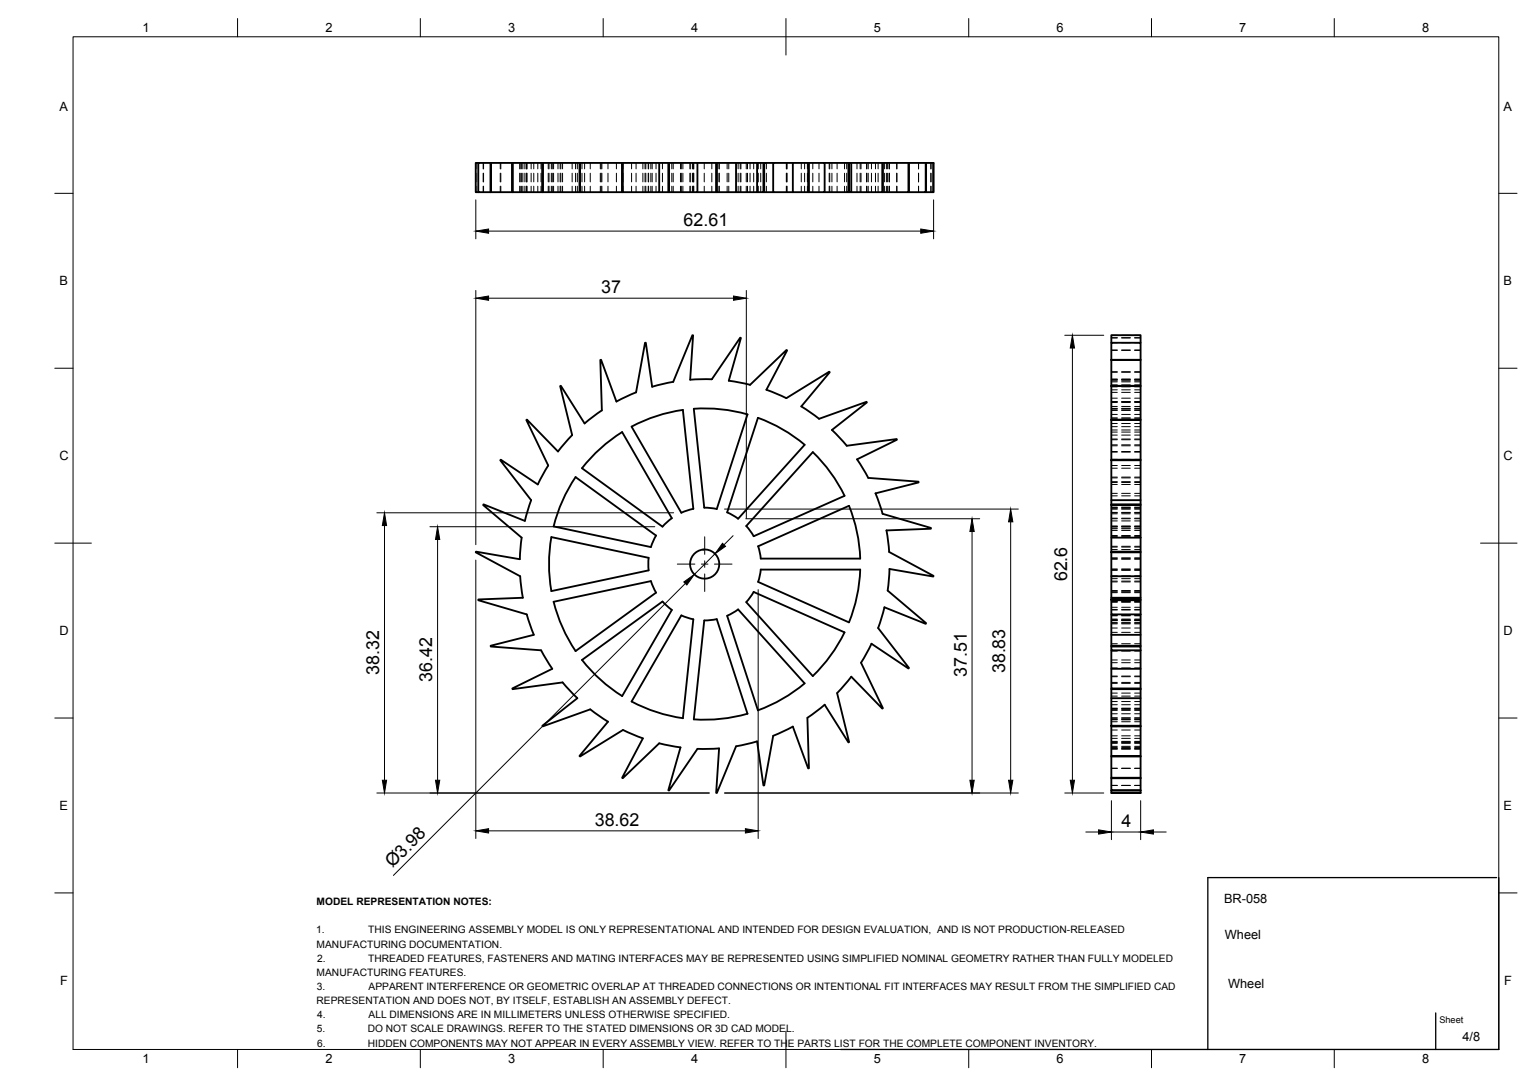
ISO-10303-21;
HEADER;
/* Generated by software containing ST-Developer
 * from STEP Tools, Inc. (www.steptools.com) 
 */

FILE_DESCRIPTION(
/* description */ (''),
/* implementation_level */ '2;1');

FILE_NAME(
/* name */ 'Wheel.step',
/* time_stamp */ '2026-10-12T16:07:47-07:00',
/* author */ (''),
/* organization */ (''),
/* preprocessor_version */ 'ST-DEVELOPER v20.2',
/* originating_system */ 'Autodesk Translation Framework v15.15.0.0',
/* authorisation */ '');

FILE_SCHEMA (('AUTOMOTIVE_DESIGN { 1 0 10303 214 3 1 1 }'));
ENDSEC;

DATA;
#10=MECHANICAL_DESIGN_GEOMETRIC_PRESENTATION_REPRESENTATION('',(#94),#8779);
#80=SHAPE_REPRESENTATION_RELATIONSHIP('SRR','None',#8809,#87);
#87=ADVANCED_BREP_SHAPE_REPRESENTATION('',(#104),#8772);
#94=STYLED_ITEM('',(#8853),#104);
#104=MANIFOLD_SOLID_BREP('Body1',#5114);
#114=FACE_BOUND('',#934,.T.);
#115=FACE_BOUND('',#935,.T.);
#116=FACE_BOUND('',#936,.T.);
#117=FACE_BOUND('',#937,.T.);
#118=FACE_BOUND('',#938,.T.);
#119=FACE_BOUND('',#939,.T.);
#120=FACE_BOUND('',#940,.T.);
#121=FACE_BOUND('',#941,.T.);
#122=FACE_BOUND('',#942,.T.);
#123=FACE_BOUND('',#943,.T.);
#124=FACE_BOUND('',#944,.T.);
#125=FACE_BOUND('',#945,.T.);
#126=FACE_BOUND('',#946,.T.);
#127=FACE_BOUND('',#947,.T.);
#128=FACE_BOUND('',#948,.T.);
#129=FACE_BOUND('',#949,.T.);
#130=FACE_BOUND('',#951,.T.);
#131=FACE_BOUND('',#952,.T.);
#132=FACE_BOUND('',#953,.T.);
#133=FACE_BOUND('',#954,.T.);
#134=FACE_BOUND('',#955,.T.);
#135=FACE_BOUND('',#956,.T.);
#136=FACE_BOUND('',#957,.T.);
#137=FACE_BOUND('',#958,.T.);
#138=FACE_BOUND('',#959,.T.);
#139=FACE_BOUND('',#960,.T.);
#140=FACE_BOUND('',#961,.T.);
#141=FACE_BOUND('',#962,.T.);
#142=FACE_BOUND('',#963,.T.);
#143=FACE_BOUND('',#964,.T.);
#144=FACE_BOUND('',#965,.T.);
#145=FACE_BOUND('',#966,.T.);
#169=CIRCLE('',#5208,25.2882678496568);
#170=CIRCLE('',#5209,25.2882678496568);
#171=CIRCLE('',#5211,25.2882678496568);
#172=CIRCLE('',#5212,25.2882678496568);
#173=CIRCLE('',#5217,25.2882678496568);
#174=CIRCLE('',#5218,25.2882678496568);
#175=CIRCLE('',#5220,25.2882678496568);
#176=CIRCLE('',#5221,25.2882678496568);
#177=CIRCLE('',#5226,25.2882678496568);
#178=CIRCLE('',#5227,25.2882678496568);
#179=CIRCLE('',#5232,25.2882678496568);
#180=CIRCLE('',#5233,25.2882678496568);
#181=CIRCLE('',#5235,25.2882678496568);
#182=CIRCLE('',#5236,25.2882678496568);
#183=CIRCLE('',#5244,25.2882678496568);
#184=CIRCLE('',#5245,25.2882678496568);
#185=CIRCLE('',#5250,25.2882678496568);
#186=CIRCLE('',#5251,25.2882678496568);
#187=CIRCLE('',#5258,21.2882678496568);
#188=CIRCLE('',#5259,21.2882678496568);
#189=CIRCLE('',#5261,21.2882678496568);
#190=CIRCLE('',#5262,21.2882678496568);
#191=CIRCLE('',#5264,7.71108476483471);
#192=CIRCLE('',#5265,7.71108476483471);
#193=CIRCLE('',#5267,7.71108476483471);
#194=CIRCLE('',#5268,7.71108476483471);
#195=CIRCLE('',#5272,21.2882678496568);
#196=CIRCLE('',#5273,21.2882678496568);
#197=CIRCLE('',#5275,7.71108476483471);
#198=CIRCLE('',#5276,7.71108476483471);
#199=CIRCLE('',#5280,21.2882678496568);
#200=CIRCLE('',#5281,21.2882678496568);
#201=CIRCLE('',#5283,7.71108476483471);
#202=CIRCLE('',#5284,7.71108476483471);
#203=CIRCLE('',#5289,25.2882678496568);
#204=CIRCLE('',#5290,25.2882678496568);
#205=CIRCLE('',#5292,25.2882678496568);
#206=CIRCLE('',#5293,25.2882678496568);
#207=CIRCLE('',#5298,25.2882678496568);
#208=CIRCLE('',#5299,25.2882678496568);
#209=CIRCLE('',#5301,25.2882678496568);
#210=CIRCLE('',#5302,25.2882678496568);
#211=CIRCLE('',#5307,25.2882678496568);
#212=CIRCLE('',#5308,25.2882678496568);
#213=CIRCLE('',#5316,25.2882678496568);
#214=CIRCLE('',#5317,25.2882678496568);
#215=CIRCLE('',#5324,21.2882678496568);
#216=CIRCLE('',#5325,21.2882678496568);
#217=CIRCLE('',#5327,21.2882678496568);
#218=CIRCLE('',#5328,21.2882678496568);
#219=CIRCLE('',#5330,7.71108476483471);
#220=CIRCLE('',#5331,7.71108476483471);
#221=CIRCLE('',#5333,7.71108476483471);
#222=CIRCLE('',#5334,7.71108476483471);
#223=CIRCLE('',#5338,21.2882678496568);
#224=CIRCLE('',#5339,21.2882678496568);
#225=CIRCLE('',#5341,7.71108476483471);
#226=CIRCLE('',#5342,7.71108476483471);
#227=CIRCLE('',#5346,21.2882678496568);
#228=CIRCLE('',#5347,21.2882678496568);
#229=CIRCLE('',#5349,21.2882678496568);
#230=CIRCLE('',#5350,21.2882678496568);
#231=CIRCLE('',#5352,7.71108476483471);
#232=CIRCLE('',#5353,7.71108476483471);
#233=CIRCLE('',#5355,7.71108476483471);
#234=CIRCLE('',#5356,7.71108476483471);
#235=CIRCLE('',#5360,21.2882678496568);
#236=CIRCLE('',#5361,21.2882678496568);
#237=CIRCLE('',#5363,21.2882678496568);
#238=CIRCLE('',#5364,21.2882678496568);
#239=CIRCLE('',#5366,7.71108476483471);
#240=CIRCLE('',#5367,7.71108476483471);
#241=CIRCLE('',#5369,7.71108476483471);
#242=CIRCLE('',#5370,7.71108476483471);
#243=CIRCLE('',#5374,21.2882678496568);
#244=CIRCLE('',#5375,21.2882678496568);
#245=CIRCLE('',#5377,7.71108476483471);
#246=CIRCLE('',#5378,7.71108476483471);
#247=CIRCLE('',#5384,21.2882678496568);
#248=CIRCLE('',#5385,21.2882678496568);
#249=CIRCLE('',#5387,7.71108476483471);
#250=CIRCLE('',#5388,7.71108476483471);
#251=CIRCLE('',#5395,25.2882678496568);
#252=CIRCLE('',#5396,25.2882678496568);
#253=CIRCLE('',#5398,25.2882678496568);
#254=CIRCLE('',#5399,25.2882678496568);
#255=CIRCLE('',#5404,25.2882678496568);
#256=CIRCLE('',#5405,25.2882678496568);
#257=CIRCLE('',#5410,25.2882678496568);
#258=CIRCLE('',#5411,25.2882678496568);
#259=CIRCLE('',#5413,25.2882678496568);
#260=CIRCLE('',#5414,25.2882678496568);
#261=CIRCLE('',#5419,25.2882678496568);
#262=CIRCLE('',#5420,25.2882678496568);
#263=CIRCLE('',#5422,25.2882678496568);
#264=CIRCLE('',#5423,25.2882678496568);
#265=CIRCLE('',#5437,25.2882678496568);
#266=CIRCLE('',#5438,25.2882678496568);
#267=CIRCLE('',#5442,21.2882678496568);
#268=CIRCLE('',#5443,21.2882678496568);
#269=CIRCLE('',#5445,7.71108476483471);
#270=CIRCLE('',#5446,7.71108476483471);
#271=CIRCLE('',#5450,21.2882678496568);
#272=CIRCLE('',#5451,21.2882678496568);
#273=CIRCLE('',#5453,7.71108476483471);
#274=CIRCLE('',#5454,7.71108476483471);
#275=CIRCLE('',#5461,25.2882678496568);
#276=CIRCLE('',#5462,25.2882678496568);
#277=CIRCLE('',#5464,25.2882678496568);
#278=CIRCLE('',#5465,25.2882678496568);
#279=CIRCLE('',#5470,25.2882678496568);
#280=CIRCLE('',#5471,25.2882678496568);
#281=CIRCLE('',#5476,25.2882678496568);
#282=CIRCLE('',#5477,25.2882678496568);
#283=CIRCLE('',#5479,25.2882678496568);
#284=CIRCLE('',#5480,25.2882678496568);
#285=CIRCLE('',#5485,25.2882678496568);
#286=CIRCLE('',#5486,25.2882678496568);
#287=CIRCLE('',#5491,25.2882678496568);
#288=CIRCLE('',#5492,25.2882678496568);
#289=CIRCLE('',#5505,1.99137169252308);
#290=CIRCLE('',#5506,1.99137169252308);
#396=CYLINDRICAL_SURFACE('',#5207,25.2882678496568);
#397=CYLINDRICAL_SURFACE('',#5210,25.2882678496568);
#398=CYLINDRICAL_SURFACE('',#5216,25.2882678496568);
#399=CYLINDRICAL_SURFACE('',#5219,25.2882678496568);
#400=CYLINDRICAL_SURFACE('',#5225,25.2882678496568);
#401=CYLINDRICAL_SURFACE('',#5231,25.2882678496568);
#402=CYLINDRICAL_SURFACE('',#5234,25.2882678496568);
#403=CYLINDRICAL_SURFACE('',#5243,25.2882678496568);
#404=CYLINDRICAL_SURFACE('',#5249,25.2882678496568);
#405=CYLINDRICAL_SURFACE('',#5257,21.2882678496568);
#406=CYLINDRICAL_SURFACE('',#5260,21.2882678496568);
#407=CYLINDRICAL_SURFACE('',#5263,7.71108476483471);
#408=CYLINDRICAL_SURFACE('',#5266,7.71108476483471);
#409=CYLINDRICAL_SURFACE('',#5271,21.2882678496568);
#410=CYLINDRICAL_SURFACE('',#5274,7.71108476483471);
#411=CYLINDRICAL_SURFACE('',#5279,21.2882678496568);
#412=CYLINDRICAL_SURFACE('',#5282,7.71108476483471);
#413=CYLINDRICAL_SURFACE('',#5288,25.2882678496568);
#414=CYLINDRICAL_SURFACE('',#5291,25.2882678496568);
#415=CYLINDRICAL_SURFACE('',#5297,25.2882678496568);
#416=CYLINDRICAL_SURFACE('',#5300,25.2882678496568);
#417=CYLINDRICAL_SURFACE('',#5306,25.2882678496568);
#418=CYLINDRICAL_SURFACE('',#5315,25.2882678496568);
#419=CYLINDRICAL_SURFACE('',#5323,21.2882678496568);
#420=CYLINDRICAL_SURFACE('',#5326,21.2882678496568);
#421=CYLINDRICAL_SURFACE('',#5329,7.71108476483471);
#422=CYLINDRICAL_SURFACE('',#5332,7.71108476483471);
#423=CYLINDRICAL_SURFACE('',#5337,21.2882678496568);
#424=CYLINDRICAL_SURFACE('',#5340,7.71108476483471);
#425=CYLINDRICAL_SURFACE('',#5345,21.2882678496568);
#426=CYLINDRICAL_SURFACE('',#5348,21.2882678496568);
#427=CYLINDRICAL_SURFACE('',#5351,7.71108476483471);
#428=CYLINDRICAL_SURFACE('',#5354,7.71108476483471);
#429=CYLINDRICAL_SURFACE('',#5359,21.2882678496568);
#430=CYLINDRICAL_SURFACE('',#5362,21.2882678496568);
#431=CYLINDRICAL_SURFACE('',#5365,7.71108476483471);
#432=CYLINDRICAL_SURFACE('',#5368,7.71108476483471);
#433=CYLINDRICAL_SURFACE('',#5373,21.2882678496568);
#434=CYLINDRICAL_SURFACE('',#5376,7.71108476483471);
#435=CYLINDRICAL_SURFACE('',#5383,21.2882678496568);
#436=CYLINDRICAL_SURFACE('',#5386,7.71108476483471);
#437=CYLINDRICAL_SURFACE('',#5394,25.2882678496568);
#438=CYLINDRICAL_SURFACE('',#5397,25.2882678496568);
#439=CYLINDRICAL_SURFACE('',#5403,25.2882678496568);
#440=CYLINDRICAL_SURFACE('',#5409,25.2882678496568);
#441=CYLINDRICAL_SURFACE('',#5412,25.2882678496568);
#442=CYLINDRICAL_SURFACE('',#5418,25.2882678496568);
#443=CYLINDRICAL_SURFACE('',#5421,25.2882678496568);
#444=CYLINDRICAL_SURFACE('',#5436,25.2882678496568);
#445=CYLINDRICAL_SURFACE('',#5441,21.2882678496568);
#446=CYLINDRICAL_SURFACE('',#5444,7.71108476483471);
#447=CYLINDRICAL_SURFACE('',#5449,21.2882678496568);
#448=CYLINDRICAL_SURFACE('',#5452,7.71108476483471);
#449=CYLINDRICAL_SURFACE('',#5460,25.2882678496568);
#450=CYLINDRICAL_SURFACE('',#5463,25.2882678496568);
#451=CYLINDRICAL_SURFACE('',#5469,25.2882678496568);
#452=CYLINDRICAL_SURFACE('',#5475,25.2882678496568);
#453=CYLINDRICAL_SURFACE('',#5478,25.2882678496568);
#454=CYLINDRICAL_SURFACE('',#5484,25.2882678496568);
#455=CYLINDRICAL_SURFACE('',#5490,25.2882678496568);
#456=CYLINDRICAL_SURFACE('',#5504,1.99137169252308);
#475=FACE_OUTER_BOUND('',#752,.T.);
#476=FACE_OUTER_BOUND('',#753,.T.);
#477=FACE_OUTER_BOUND('',#754,.T.);
#478=FACE_OUTER_BOUND('',#755,.T.);
#479=FACE_OUTER_BOUND('',#756,.T.);
#480=FACE_OUTER_BOUND('',#757,.T.);
#481=FACE_OUTER_BOUND('',#758,.T.);
#482=FACE_OUTER_BOUND('',#759,.T.);
#483=FACE_OUTER_BOUND('',#760,.T.);
#484=FACE_OUTER_BOUND('',#761,.T.);
#485=FACE_OUTER_BOUND('',#762,.T.);
#486=FACE_OUTER_BOUND('',#763,.T.);
#487=FACE_OUTER_BOUND('',#764,.T.);
#488=FACE_OUTER_BOUND('',#765,.T.);
#489=FACE_OUTER_BOUND('',#766,.T.);
#490=FACE_OUTER_BOUND('',#767,.T.);
#491=FACE_OUTER_BOUND('',#768,.T.);
#492=FACE_OUTER_BOUND('',#769,.T.);
#493=FACE_OUTER_BOUND('',#770,.T.);
#494=FACE_OUTER_BOUND('',#771,.T.);
#495=FACE_OUTER_BOUND('',#772,.T.);
#496=FACE_OUTER_BOUND('',#773,.T.);
#497=FACE_OUTER_BOUND('',#774,.T.);
#498=FACE_OUTER_BOUND('',#775,.T.);
#499=FACE_OUTER_BOUND('',#776,.T.);
#500=FACE_OUTER_BOUND('',#777,.T.);
#501=FACE_OUTER_BOUND('',#778,.T.);
#502=FACE_OUTER_BOUND('',#779,.T.);
#503=FACE_OUTER_BOUND('',#780,.T.);
#504=FACE_OUTER_BOUND('',#781,.T.);
#505=FACE_OUTER_BOUND('',#782,.T.);
#506=FACE_OUTER_BOUND('',#783,.T.);
#507=FACE_OUTER_BOUND('',#784,.T.);
#508=FACE_OUTER_BOUND('',#785,.T.);
#509=FACE_OUTER_BOUND('',#786,.T.);
#510=FACE_OUTER_BOUND('',#787,.T.);
#511=FACE_OUTER_BOUND('',#788,.T.);
#512=FACE_OUTER_BOUND('',#789,.T.);
#513=FACE_OUTER_BOUND('',#790,.T.);
#514=FACE_OUTER_BOUND('',#791,.T.);
#515=FACE_OUTER_BOUND('',#792,.T.);
#516=FACE_OUTER_BOUND('',#793,.T.);
#517=FACE_OUTER_BOUND('',#794,.T.);
#518=FACE_OUTER_BOUND('',#795,.T.);
#519=FACE_OUTER_BOUND('',#796,.T.);
#520=FACE_OUTER_BOUND('',#797,.T.);
#521=FACE_OUTER_BOUND('',#798,.T.);
#522=FACE_OUTER_BOUND('',#799,.T.);
#523=FACE_OUTER_BOUND('',#800,.T.);
#524=FACE_OUTER_BOUND('',#801,.T.);
#525=FACE_OUTER_BOUND('',#802,.T.);
#526=FACE_OUTER_BOUND('',#803,.T.);
#527=FACE_OUTER_BOUND('',#804,.T.);
#528=FACE_OUTER_BOUND('',#805,.T.);
#529=FACE_OUTER_BOUND('',#806,.T.);
#530=FACE_OUTER_BOUND('',#807,.T.);
#531=FACE_OUTER_BOUND('',#808,.T.);
#532=FACE_OUTER_BOUND('',#809,.T.);
#533=FACE_OUTER_BOUND('',#810,.T.);
#534=FACE_OUTER_BOUND('',#811,.T.);
#535=FACE_OUTER_BOUND('',#812,.T.);
#536=FACE_OUTER_BOUND('',#813,.T.);
#537=FACE_OUTER_BOUND('',#814,.T.);
#538=FACE_OUTER_BOUND('',#815,.T.);
#539=FACE_OUTER_BOUND('',#816,.T.);
#540=FACE_OUTER_BOUND('',#817,.T.);
#541=FACE_OUTER_BOUND('',#818,.T.);
#542=FACE_OUTER_BOUND('',#819,.T.);
#543=FACE_OUTER_BOUND('',#820,.T.);
#544=FACE_OUTER_BOUND('',#821,.T.);
#545=FACE_OUTER_BOUND('',#822,.T.);
#546=FACE_OUTER_BOUND('',#823,.T.);
#547=FACE_OUTER_BOUND('',#824,.T.);
#548=FACE_OUTER_BOUND('',#825,.T.);
#549=FACE_OUTER_BOUND('',#826,.T.);
#550=FACE_OUTER_BOUND('',#827,.T.);
#551=FACE_OUTER_BOUND('',#828,.T.);
#552=FACE_OUTER_BOUND('',#829,.T.);
#553=FACE_OUTER_BOUND('',#830,.T.);
#554=FACE_OUTER_BOUND('',#831,.T.);
#555=FACE_OUTER_BOUND('',#832,.T.);
#556=FACE_OUTER_BOUND('',#833,.T.);
#557=FACE_OUTER_BOUND('',#834,.T.);
#558=FACE_OUTER_BOUND('',#835,.T.);
#559=FACE_OUTER_BOUND('',#836,.T.);
#560=FACE_OUTER_BOUND('',#837,.T.);
#561=FACE_OUTER_BOUND('',#838,.T.);
#562=FACE_OUTER_BOUND('',#839,.T.);
#563=FACE_OUTER_BOUND('',#840,.T.);
#564=FACE_OUTER_BOUND('',#841,.T.);
#565=FACE_OUTER_BOUND('',#842,.T.);
#566=FACE_OUTER_BOUND('',#843,.T.);
#567=FACE_OUTER_BOUND('',#844,.T.);
#568=FACE_OUTER_BOUND('',#845,.T.);
#569=FACE_OUTER_BOUND('',#846,.T.);
#570=FACE_OUTER_BOUND('',#847,.T.);
#571=FACE_OUTER_BOUND('',#848,.T.);
#572=FACE_OUTER_BOUND('',#849,.T.);
#573=FACE_OUTER_BOUND('',#850,.T.);
#574=FACE_OUTER_BOUND('',#851,.T.);
#575=FACE_OUTER_BOUND('',#852,.T.);
#576=FACE_OUTER_BOUND('',#853,.T.);
#577=FACE_OUTER_BOUND('',#854,.T.);
#578=FACE_OUTER_BOUND('',#855,.T.);
#579=FACE_OUTER_BOUND('',#856,.T.);
#580=FACE_OUTER_BOUND('',#857,.T.);
#581=FACE_OUTER_BOUND('',#858,.T.);
#582=FACE_OUTER_BOUND('',#859,.T.);
#583=FACE_OUTER_BOUND('',#860,.T.);
#584=FACE_OUTER_BOUND('',#861,.T.);
#585=FACE_OUTER_BOUND('',#862,.T.);
#586=FACE_OUTER_BOUND('',#863,.T.);
#587=FACE_OUTER_BOUND('',#864,.T.);
#588=FACE_OUTER_BOUND('',#865,.T.);
#589=FACE_OUTER_BOUND('',#866,.T.);
#590=FACE_OUTER_BOUND('',#867,.T.);
#591=FACE_OUTER_BOUND('',#868,.T.);
#592=FACE_OUTER_BOUND('',#869,.T.);
#593=FACE_OUTER_BOUND('',#870,.T.);
#594=FACE_OUTER_BOUND('',#871,.T.);
#595=FACE_OUTER_BOUND('',#872,.T.);
#596=FACE_OUTER_BOUND('',#873,.T.);
#597=FACE_OUTER_BOUND('',#874,.T.);
#598=FACE_OUTER_BOUND('',#875,.T.);
#599=FACE_OUTER_BOUND('',#876,.T.);
#600=FACE_OUTER_BOUND('',#877,.T.);
#601=FACE_OUTER_BOUND('',#878,.T.);
#602=FACE_OUTER_BOUND('',#879,.T.);
#603=FACE_OUTER_BOUND('',#880,.T.);
#604=FACE_OUTER_BOUND('',#881,.T.);
#605=FACE_OUTER_BOUND('',#882,.T.);
#606=FACE_OUTER_BOUND('',#883,.T.);
#607=FACE_OUTER_BOUND('',#884,.T.);
#608=FACE_OUTER_BOUND('',#885,.T.);
#609=FACE_OUTER_BOUND('',#886,.T.);
#610=FACE_OUTER_BOUND('',#887,.T.);
#611=FACE_OUTER_BOUND('',#888,.T.);
#612=FACE_OUTER_BOUND('',#889,.T.);
#613=FACE_OUTER_BOUND('',#890,.T.);
#614=FACE_OUTER_BOUND('',#891,.T.);
#615=FACE_OUTER_BOUND('',#892,.T.);
#616=FACE_OUTER_BOUND('',#893,.T.);
#617=FACE_OUTER_BOUND('',#894,.T.);
#618=FACE_OUTER_BOUND('',#895,.T.);
#619=FACE_OUTER_BOUND('',#896,.T.);
#620=FACE_OUTER_BOUND('',#897,.T.);
#621=FACE_OUTER_BOUND('',#898,.T.);
#622=FACE_OUTER_BOUND('',#899,.T.);
#623=FACE_OUTER_BOUND('',#900,.T.);
#624=FACE_OUTER_BOUND('',#901,.T.);
#625=FACE_OUTER_BOUND('',#902,.T.);
#626=FACE_OUTER_BOUND('',#903,.T.);
#627=FACE_OUTER_BOUND('',#904,.T.);
#628=FACE_OUTER_BOUND('',#905,.T.);
#629=FACE_OUTER_BOUND('',#906,.T.);
#630=FACE_OUTER_BOUND('',#907,.T.);
#631=FACE_OUTER_BOUND('',#908,.T.);
#632=FACE_OUTER_BOUND('',#909,.T.);
#633=FACE_OUTER_BOUND('',#910,.T.);
#634=FACE_OUTER_BOUND('',#911,.T.);
#635=FACE_OUTER_BOUND('',#912,.T.);
#636=FACE_OUTER_BOUND('',#913,.T.);
#637=FACE_OUTER_BOUND('',#914,.T.);
#638=FACE_OUTER_BOUND('',#915,.T.);
#639=FACE_OUTER_BOUND('',#916,.T.);
#640=FACE_OUTER_BOUND('',#917,.T.);
#641=FACE_OUTER_BOUND('',#918,.T.);
#642=FACE_OUTER_BOUND('',#919,.T.);
#643=FACE_OUTER_BOUND('',#920,.T.);
#644=FACE_OUTER_BOUND('',#921,.T.);
#645=FACE_OUTER_BOUND('',#922,.T.);
#646=FACE_OUTER_BOUND('',#923,.T.);
#647=FACE_OUTER_BOUND('',#924,.T.);
#648=FACE_OUTER_BOUND('',#925,.T.);
#649=FACE_OUTER_BOUND('',#926,.T.);
#650=FACE_OUTER_BOUND('',#927,.T.);
#651=FACE_OUTER_BOUND('',#928,.T.);
#652=FACE_OUTER_BOUND('',#929,.T.);
#653=FACE_OUTER_BOUND('',#930,.T.);
#654=FACE_OUTER_BOUND('',#931,.T.);
#655=FACE_OUTER_BOUND('',#932,.T.);
#656=FACE_OUTER_BOUND('',#933,.T.);
#657=FACE_OUTER_BOUND('',#950,.T.);
#752=EDGE_LOOP('',(#3240,#3241,#3242,#3243));
#753=EDGE_LOOP('',(#3244,#3245,#3246,#3247));
#754=EDGE_LOOP('',(#3248,#3249,#3250,#3251));
#755=EDGE_LOOP('',(#3252,#3253,#3254,#3255));
#756=EDGE_LOOP('',(#3256,#3257,#3258,#3259));
#757=EDGE_LOOP('',(#3260,#3261,#3262,#3263));
#758=EDGE_LOOP('',(#3264,#3265,#3266,#3267));
#759=EDGE_LOOP('',(#3268,#3269,#3270,#3271));
#760=EDGE_LOOP('',(#3272,#3273,#3274,#3275));
#761=EDGE_LOOP('',(#3276,#3277,#3278,#3279));
#762=EDGE_LOOP('',(#3280,#3281,#3282,#3283));
#763=EDGE_LOOP('',(#3284,#3285,#3286,#3287));
#764=EDGE_LOOP('',(#3288,#3289,#3290,#3291));
#765=EDGE_LOOP('',(#3292,#3293,#3294,#3295));
#766=EDGE_LOOP('',(#3296,#3297,#3298,#3299));
#767=EDGE_LOOP('',(#3300,#3301,#3302,#3303));
#768=EDGE_LOOP('',(#3304,#3305,#3306,#3307));
#769=EDGE_LOOP('',(#3308,#3309,#3310,#3311));
#770=EDGE_LOOP('',(#3312,#3313,#3314,#3315));
#771=EDGE_LOOP('',(#3316,#3317,#3318,#3319));
#772=EDGE_LOOP('',(#3320,#3321,#3322,#3323));
#773=EDGE_LOOP('',(#3324,#3325,#3326,#3327));
#774=EDGE_LOOP('',(#3328,#3329,#3330,#3331));
#775=EDGE_LOOP('',(#3332,#3333,#3334,#3335));
#776=EDGE_LOOP('',(#3336,#3337,#3338,#3339));
#777=EDGE_LOOP('',(#3340,#3341,#3342,#3343));
#778=EDGE_LOOP('',(#3344,#3345,#3346,#3347));
#779=EDGE_LOOP('',(#3348,#3349,#3350,#3351));
#780=EDGE_LOOP('',(#3352,#3353,#3354,#3355));
#781=EDGE_LOOP('',(#3356,#3357,#3358,#3359));
#782=EDGE_LOOP('',(#3360,#3361,#3362,#3363));
#783=EDGE_LOOP('',(#3364,#3365,#3366,#3367));
#784=EDGE_LOOP('',(#3368,#3369,#3370,#3371));
#785=EDGE_LOOP('',(#3372,#3373,#3374,#3375));
#786=EDGE_LOOP('',(#3376,#3377,#3378,#3379));
#787=EDGE_LOOP('',(#3380,#3381,#3382,#3383));
#788=EDGE_LOOP('',(#3384,#3385,#3386,#3387));
#789=EDGE_LOOP('',(#3388,#3389,#3390,#3391));
#790=EDGE_LOOP('',(#3392,#3393,#3394,#3395));
#791=EDGE_LOOP('',(#3396,#3397,#3398,#3399));
#792=EDGE_LOOP('',(#3400,#3401,#3402,#3403));
#793=EDGE_LOOP('',(#3404,#3405,#3406,#3407));
#794=EDGE_LOOP('',(#3408,#3409,#3410,#3411));
#795=EDGE_LOOP('',(#3412,#3413,#3414,#3415));
#796=EDGE_LOOP('',(#3416,#3417,#3418,#3419));
#797=EDGE_LOOP('',(#3420,#3421,#3422,#3423));
#798=EDGE_LOOP('',(#3424,#3425,#3426,#3427));
#799=EDGE_LOOP('',(#3428,#3429,#3430,#3431));
#800=EDGE_LOOP('',(#3432,#3433,#3434,#3435));
#801=EDGE_LOOP('',(#3436,#3437,#3438,#3439));
#802=EDGE_LOOP('',(#3440,#3441,#3442,#3443));
#803=EDGE_LOOP('',(#3444,#3445,#3446,#3447));
#804=EDGE_LOOP('',(#3448,#3449,#3450,#3451));
#805=EDGE_LOOP('',(#3452,#3453,#3454,#3455));
#806=EDGE_LOOP('',(#3456,#3457,#3458,#3459));
#807=EDGE_LOOP('',(#3460,#3461,#3462,#3463));
#808=EDGE_LOOP('',(#3464,#3465,#3466,#3467));
#809=EDGE_LOOP('',(#3468,#3469,#3470,#3471));
#810=EDGE_LOOP('',(#3472,#3473,#3474,#3475));
#811=EDGE_LOOP('',(#3476,#3477,#3478,#3479));
#812=EDGE_LOOP('',(#3480,#3481,#3482,#3483));
#813=EDGE_LOOP('',(#3484,#3485,#3486,#3487));
#814=EDGE_LOOP('',(#3488,#3489,#3490,#3491));
#815=EDGE_LOOP('',(#3492,#3493,#3494,#3495));
#816=EDGE_LOOP('',(#3496,#3497,#3498,#3499));
#817=EDGE_LOOP('',(#3500,#3501,#3502,#3503));
#818=EDGE_LOOP('',(#3504,#3505,#3506,#3507));
#819=EDGE_LOOP('',(#3508,#3509,#3510,#3511));
#820=EDGE_LOOP('',(#3512,#3513,#3514,#3515));
#821=EDGE_LOOP('',(#3516,#3517,#3518,#3519));
#822=EDGE_LOOP('',(#3520,#3521,#3522,#3523));
#823=EDGE_LOOP('',(#3524,#3525,#3526,#3527));
#824=EDGE_LOOP('',(#3528,#3529,#3530,#3531));
#825=EDGE_LOOP('',(#3532,#3533,#3534,#3535));
#826=EDGE_LOOP('',(#3536,#3537,#3538,#3539));
#827=EDGE_LOOP('',(#3540,#3541,#3542,#3543));
#828=EDGE_LOOP('',(#3544,#3545,#3546,#3547));
#829=EDGE_LOOP('',(#3548,#3549,#3550,#3551));
#830=EDGE_LOOP('',(#3552,#3553,#3554,#3555));
#831=EDGE_LOOP('',(#3556,#3557,#3558,#3559));
#832=EDGE_LOOP('',(#3560,#3561,#3562,#3563));
#833=EDGE_LOOP('',(#3564,#3565,#3566,#3567));
#834=EDGE_LOOP('',(#3568,#3569,#3570,#3571));
#835=EDGE_LOOP('',(#3572,#3573,#3574,#3575));
#836=EDGE_LOOP('',(#3576,#3577,#3578,#3579));
#837=EDGE_LOOP('',(#3580,#3581,#3582,#3583));
#838=EDGE_LOOP('',(#3584,#3585,#3586,#3587));
#839=EDGE_LOOP('',(#3588,#3589,#3590,#3591));
#840=EDGE_LOOP('',(#3592,#3593,#3594,#3595));
#841=EDGE_LOOP('',(#3596,#3597,#3598,#3599));
#842=EDGE_LOOP('',(#3600,#3601,#3602,#3603));
#843=EDGE_LOOP('',(#3604,#3605,#3606,#3607));
#844=EDGE_LOOP('',(#3608,#3609,#3610,#3611));
#845=EDGE_LOOP('',(#3612,#3613,#3614,#3615));
#846=EDGE_LOOP('',(#3616,#3617,#3618,#3619));
#847=EDGE_LOOP('',(#3620,#3621,#3622,#3623));
#848=EDGE_LOOP('',(#3624,#3625,#3626,#3627));
#849=EDGE_LOOP('',(#3628,#3629,#3630,#3631));
#850=EDGE_LOOP('',(#3632,#3633,#3634,#3635));
#851=EDGE_LOOP('',(#3636,#3637,#3638,#3639));
#852=EDGE_LOOP('',(#3640,#3641,#3642,#3643));
#853=EDGE_LOOP('',(#3644,#3645,#3646,#3647));
#854=EDGE_LOOP('',(#3648,#3649,#3650,#3651));
#855=EDGE_LOOP('',(#3652,#3653,#3654,#3655));
#856=EDGE_LOOP('',(#3656,#3657,#3658,#3659));
#857=EDGE_LOOP('',(#3660,#3661,#3662,#3663));
#858=EDGE_LOOP('',(#3664,#3665,#3666,#3667));
#859=EDGE_LOOP('',(#3668,#3669,#3670,#3671));
#860=EDGE_LOOP('',(#3672,#3673,#3674,#3675));
#861=EDGE_LOOP('',(#3676,#3677,#3678,#3679));
#862=EDGE_LOOP('',(#3680,#3681,#3682,#3683));
#863=EDGE_LOOP('',(#3684,#3685,#3686,#3687));
#864=EDGE_LOOP('',(#3688,#3689,#3690,#3691));
#865=EDGE_LOOP('',(#3692,#3693,#3694,#3695));
#866=EDGE_LOOP('',(#3696,#3697,#3698,#3699));
#867=EDGE_LOOP('',(#3700,#3701,#3702,#3703));
#868=EDGE_LOOP('',(#3704,#3705,#3706,#3707));
#869=EDGE_LOOP('',(#3708,#3709,#3710,#3711));
#870=EDGE_LOOP('',(#3712,#3713,#3714,#3715));
#871=EDGE_LOOP('',(#3716,#3717,#3718,#3719));
#872=EDGE_LOOP('',(#3720,#3721,#3722,#3723));
#873=EDGE_LOOP('',(#3724,#3725,#3726,#3727));
#874=EDGE_LOOP('',(#3728,#3729,#3730,#3731));
#875=EDGE_LOOP('',(#3732,#3733,#3734,#3735));
#876=EDGE_LOOP('',(#3736,#3737,#3738,#3739));
#877=EDGE_LOOP('',(#3740,#3741,#3742,#3743));
#878=EDGE_LOOP('',(#3744,#3745,#3746,#3747));
#879=EDGE_LOOP('',(#3748,#3749,#3750,#3751));
#880=EDGE_LOOP('',(#3752,#3753,#3754,#3755));
#881=EDGE_LOOP('',(#3756,#3757,#3758,#3759));
#882=EDGE_LOOP('',(#3760,#3761,#3762,#3763));
#883=EDGE_LOOP('',(#3764,#3765,#3766,#3767));
#884=EDGE_LOOP('',(#3768,#3769,#3770,#3771));
#885=EDGE_LOOP('',(#3772,#3773,#3774,#3775));
#886=EDGE_LOOP('',(#3776,#3777,#3778,#3779));
#887=EDGE_LOOP('',(#3780,#3781,#3782,#3783));
#888=EDGE_LOOP('',(#3784,#3785,#3786,#3787));
#889=EDGE_LOOP('',(#3788,#3789,#3790,#3791));
#890=EDGE_LOOP('',(#3792,#3793,#3794,#3795));
#891=EDGE_LOOP('',(#3796,#3797,#3798,#3799));
#892=EDGE_LOOP('',(#3800,#3801,#3802,#3803));
#893=EDGE_LOOP('',(#3804,#3805,#3806,#3807));
#894=EDGE_LOOP('',(#3808,#3809,#3810,#3811));
#895=EDGE_LOOP('',(#3812,#3813,#3814,#3815));
#896=EDGE_LOOP('',(#3816,#3817,#3818,#3819));
#897=EDGE_LOOP('',(#3820,#3821,#3822,#3823));
#898=EDGE_LOOP('',(#3824,#3825,#3826,#3827));
#899=EDGE_LOOP('',(#3828,#3829,#3830,#3831));
#900=EDGE_LOOP('',(#3832,#3833,#3834,#3835));
#901=EDGE_LOOP('',(#3836,#3837,#3838,#3839));
#902=EDGE_LOOP('',(#3840,#3841,#3842,#3843));
#903=EDGE_LOOP('',(#3844,#3845,#3846,#3847));
#904=EDGE_LOOP('',(#3848,#3849,#3850,#3851));
#905=EDGE_LOOP('',(#3852,#3853,#3854,#3855));
#906=EDGE_LOOP('',(#3856,#3857,#3858,#3859));
#907=EDGE_LOOP('',(#3860,#3861,#3862,#3863));
#908=EDGE_LOOP('',(#3864,#3865,#3866,#3867));
#909=EDGE_LOOP('',(#3868,#3869,#3870,#3871));
#910=EDGE_LOOP('',(#3872,#3873,#3874,#3875));
#911=EDGE_LOOP('',(#3876,#3877,#3878,#3879));
#912=EDGE_LOOP('',(#3880,#3881,#3882,#3883));
#913=EDGE_LOOP('',(#3884,#3885,#3886,#3887));
#914=EDGE_LOOP('',(#3888,#3889,#3890,#3891));
#915=EDGE_LOOP('',(#3892,#3893,#3894,#3895));
#916=EDGE_LOOP('',(#3896,#3897,#3898,#3899));
#917=EDGE_LOOP('',(#3900,#3901,#3902,#3903));
#918=EDGE_LOOP('',(#3904,#3905,#3906,#3907));
#919=EDGE_LOOP('',(#3908,#3909,#3910,#3911));
#920=EDGE_LOOP('',(#3912,#3913,#3914,#3915));
#921=EDGE_LOOP('',(#3916,#3917,#3918,#3919));
#922=EDGE_LOOP('',(#3920,#3921,#3922,#3923));
#923=EDGE_LOOP('',(#3924,#3925,#3926,#3927));
#924=EDGE_LOOP('',(#3928,#3929,#3930,#3931));
#925=EDGE_LOOP('',(#3932,#3933,#3934,#3935));
#926=EDGE_LOOP('',(#3936,#3937,#3938,#3939));
#927=EDGE_LOOP('',(#3940,#3941,#3942,#3943));
#928=EDGE_LOOP('',(#3944,#3945,#3946,#3947));
#929=EDGE_LOOP('',(#3948,#3949,#3950,#3951));
#930=EDGE_LOOP('',(#3952,#3953,#3954,#3955));
#931=EDGE_LOOP('',(#3956,#3957,#3958,#3959));
#932=EDGE_LOOP('',(#3960,#3961,#3962,#3963));
#933=EDGE_LOOP('',(#3964,#3965,#3966,#3967,#3968,#3969,#3970,#3971,#3972,
#3973,#3974,#3975,#3976,#3977,#3978,#3979,#3980,#3981,#3982,#3983,#3984,
#3985,#3986,#3987,#3988,#3989,#3990,#3991,#3992,#3993,#3994,#3995,#3996,
#3997,#3998,#3999,#4000,#4001,#4002,#4003,#4004,#4005,#4006,#4007,#4008,
#4009,#4010,#4011,#4012,#4013,#4014,#4015,#4016,#4017,#4018,#4019,#4020,
#4021,#4022,#4023,#4024,#4025,#4026,#4027,#4028,#4029,#4030,#4031,#4032,
#4033,#4034,#4035,#4036,#4037,#4038,#4039,#4040,#4041,#4042,#4043,#4044,
#4045,#4046,#4047,#4048,#4049,#4050,#4051,#4052,#4053,#4054,#4055,#4056,
#4057,#4058,#4059,#4060,#4061,#4062,#4063,#4064,#4065,#4066,#4067,#4068,
#4069,#4070,#4071,#4072,#4073,#4074,#4075,#4076,#4077,#4078,#4079,#4080,
#4081,#4082,#4083));
#934=EDGE_LOOP('',(#4084,#4085,#4086,#4087));
#935=EDGE_LOOP('',(#4088,#4089,#4090,#4091));
#936=EDGE_LOOP('',(#4092,#4093,#4094,#4095));
#937=EDGE_LOOP('',(#4096,#4097,#4098,#4099));
#938=EDGE_LOOP('',(#4100,#4101,#4102,#4103));
#939=EDGE_LOOP('',(#4104,#4105,#4106,#4107));
#940=EDGE_LOOP('',(#4108,#4109,#4110,#4111));
#941=EDGE_LOOP('',(#4112,#4113,#4114,#4115));
#942=EDGE_LOOP('',(#4116,#4117,#4118,#4119));
#943=EDGE_LOOP('',(#4120,#4121,#4122,#4123));
#944=EDGE_LOOP('',(#4124,#4125,#4126,#4127));
#945=EDGE_LOOP('',(#4128,#4129,#4130,#4131));
#946=EDGE_LOOP('',(#4132,#4133,#4134,#4135));
#947=EDGE_LOOP('',(#4136,#4137,#4138,#4139));
#948=EDGE_LOOP('',(#4140));
#949=EDGE_LOOP('',(#4141,#4142,#4143,#4144));
#950=EDGE_LOOP('',(#4145,#4146,#4147,#4148,#4149,#4150,#4151,#4152,#4153,
#4154,#4155,#4156,#4157,#4158,#4159,#4160,#4161,#4162,#4163,#4164,#4165,
#4166,#4167,#4168,#4169,#4170,#4171,#4172,#4173,#4174,#4175,#4176,#4177,
#4178,#4179,#4180,#4181,#4182,#4183,#4184,#4185,#4186,#4187,#4188,#4189,
#4190,#4191,#4192,#4193,#4194,#4195,#4196,#4197,#4198,#4199,#4200,#4201,
#4202,#4203,#4204,#4205,#4206,#4207,#4208,#4209,#4210,#4211,#4212,#4213,
#4214,#4215,#4216,#4217,#4218,#4219,#4220,#4221,#4222,#4223,#4224,#4225,
#4226,#4227,#4228,#4229,#4230,#4231,#4232,#4233,#4234,#4235,#4236,#4237,
#4238,#4239,#4240,#4241,#4242,#4243,#4244,#4245,#4246,#4247,#4248,#4249,
#4250,#4251,#4252,#4253,#4254,#4255,#4256,#4257,#4258,#4259,#4260,#4261,
#4262,#4263,#4264));
#951=EDGE_LOOP('',(#4265,#4266,#4267,#4268));
#952=EDGE_LOOP('',(#4269,#4270,#4271,#4272));
#953=EDGE_LOOP('',(#4273,#4274,#4275,#4276));
#954=EDGE_LOOP('',(#4277,#4278,#4279,#4280));
#955=EDGE_LOOP('',(#4281,#4282,#4283,#4284));
#956=EDGE_LOOP('',(#4285,#4286,#4287,#4288));
#957=EDGE_LOOP('',(#4289,#4290,#4291,#4292));
#958=EDGE_LOOP('',(#4293,#4294,#4295,#4296));
#959=EDGE_LOOP('',(#4297,#4298,#4299,#4300));
#960=EDGE_LOOP('',(#4301,#4302,#4303,#4304));
#961=EDGE_LOOP('',(#4305,#4306,#4307,#4308));
#962=EDGE_LOOP('',(#4309,#4310,#4311,#4312));
#963=EDGE_LOOP('',(#4313,#4314,#4315,#4316));
#964=EDGE_LOOP('',(#4317,#4318,#4319,#4320));
#965=EDGE_LOOP('',(#4321));
#966=EDGE_LOOP('',(#4322,#4323,#4324,#4325));
#1084=LINE('',#7252,#1569);
#1085=LINE('',#7254,#1570);
#1086=LINE('',#7256,#1571);
#1087=LINE('',#7257,#1572);
#1088=LINE('',#7260,#1573);
#1089=LINE('',#7262,#1574);
#1090=LINE('',#7263,#1575);
#1091=LINE('',#7266,#1576);
#1092=LINE('',#7268,#1577);
#1093=LINE('',#7269,#1578);
#1094=LINE('',#7274,#1579);
#1095=LINE('',#7280,#1580);
#1096=LINE('',#7285,#1581);
#1097=LINE('',#7287,#1582);
#1098=LINE('',#7289,#1583);
#1099=LINE('',#7290,#1584);
#1100=LINE('',#7293,#1585);
#1101=LINE('',#7295,#1586);
#1102=LINE('',#7296,#1587);
#1103=LINE('',#7299,#1588);
#1104=LINE('',#7301,#1589);
#1105=LINE('',#7302,#1590);
#1106=LINE('',#7307,#1591);
#1107=LINE('',#7313,#1592);
#1108=LINE('',#7317,#1593);
#1109=LINE('',#7319,#1594);
#1110=LINE('',#7320,#1595);
#1111=LINE('',#7323,#1596);
#1112=LINE('',#7325,#1597);
#1113=LINE('',#7326,#1598);
#1114=LINE('',#7329,#1599);
#1115=LINE('',#7331,#1600);
#1116=LINE('',#7332,#1601);
#1117=LINE('',#7337,#1602);
#1118=LINE('',#7342,#1603);
#1119=LINE('',#7344,#1604);
#1120=LINE('',#7346,#1605);
#1121=LINE('',#7347,#1606);
#1122=LINE('',#7350,#1607);
#1123=LINE('',#7352,#1608);
#1124=LINE('',#7353,#1609);
#1125=LINE('',#7356,#1610);
#1126=LINE('',#7358,#1611);
#1127=LINE('',#7359,#1612);
#1128=LINE('',#7364,#1613);
#1129=LINE('',#7370,#1614);
#1130=LINE('',#7374,#1615);
#1131=LINE('',#7376,#1616);
#1132=LINE('',#7377,#1617);
#1133=LINE('',#7380,#1618);
#1134=LINE('',#7382,#1619);
#1135=LINE('',#7383,#1620);
#1136=LINE('',#7385,#1621);
#1137=LINE('',#7386,#1622);
#1138=LINE('',#7389,#1623);
#1139=LINE('',#7391,#1624);
#1140=LINE('',#7392,#1625);
#1141=LINE('',#7395,#1626);
#1142=LINE('',#7397,#1627);
#1143=LINE('',#7398,#1628);
#1144=LINE('',#7401,#1629);
#1145=LINE('',#7403,#1630);
#1146=LINE('',#7404,#1631);
#1147=LINE('',#7409,#1632);
#1148=LINE('',#7414,#1633);
#1149=LINE('',#7416,#1634);
#1150=LINE('',#7418,#1635);
#1151=LINE('',#7419,#1636);
#1152=LINE('',#7422,#1637);
#1153=LINE('',#7424,#1638);
#1154=LINE('',#7425,#1639);
#1155=LINE('',#7427,#1640);
#1156=LINE('',#7428,#1641);
#1157=LINE('',#7433,#1642);
#1158=LINE('',#7437,#1643);
#1159=LINE('',#7439,#1644);
#1160=LINE('',#7440,#1645);
#1161=LINE('',#7443,#1646);
#1162=LINE('',#7445,#1647);
#1163=LINE('',#7446,#1648);
#1164=LINE('',#7448,#1649);
#1165=LINE('',#7449,#1650);
#1166=LINE('',#7453,#1651);
#1167=LINE('',#7455,#1652);
#1168=LINE('',#7457,#1653);
#1169=LINE('',#7458,#1654);
#1170=LINE('',#7462,#1655);
#1171=LINE('',#7464,#1656);
#1172=LINE('',#7466,#1657);
#1173=LINE('',#7467,#1658);
#1174=LINE('',#7472,#1659);
#1175=LINE('',#7478,#1660);
#1176=LINE('',#7484,#1661);
#1177=LINE('',#7490,#1662);
#1178=LINE('',#7493,#1663);
#1179=LINE('',#7494,#1664);
#1180=LINE('',#7498,#1665);
#1181=LINE('',#7500,#1666);
#1182=LINE('',#7502,#1667);
#1183=LINE('',#7503,#1668);
#1184=LINE('',#7508,#1669);
#1185=LINE('',#7514,#1670);
#1186=LINE('',#7519,#1671);
#1187=LINE('',#7521,#1672);
#1188=LINE('',#7523,#1673);
#1189=LINE('',#7524,#1674);
#1190=LINE('',#7526,#1675);
#1191=LINE('',#7527,#1676);
#1192=LINE('',#7532,#1677);
#1193=LINE('',#7538,#1678);
#1194=LINE('',#7543,#1679);
#1195=LINE('',#7545,#1680);
#1196=LINE('',#7547,#1681);
#1197=LINE('',#7548,#1682);
#1198=LINE('',#7551,#1683);
#1199=LINE('',#7553,#1684);
#1200=LINE('',#7554,#1685);
#1201=LINE('',#7557,#1686);
#1202=LINE('',#7559,#1687);
#1203=LINE('',#7560,#1688);
#1204=LINE('',#7565,#1689);
#1205=LINE('',#7571,#1690);
#1206=LINE('',#7576,#1691);
#1207=LINE('',#7578,#1692);
#1208=LINE('',#7580,#1693);
#1209=LINE('',#7581,#1694);
#1210=LINE('',#7584,#1695);
#1211=LINE('',#7586,#1696);
#1212=LINE('',#7587,#1697);
#1213=LINE('',#7590,#1698);
#1214=LINE('',#7592,#1699);
#1215=LINE('',#7593,#1700);
#1216=LINE('',#7598,#1701);
#1217=LINE('',#7604,#1702);
#1218=LINE('',#7608,#1703);
#1219=LINE('',#7610,#1704);
#1220=LINE('',#7611,#1705);
#1221=LINE('',#7614,#1706);
#1222=LINE('',#7616,#1707);
#1223=LINE('',#7617,#1708);
#1224=LINE('',#7620,#1709);
#1225=LINE('',#7622,#1710);
#1226=LINE('',#7623,#1711);
#1227=LINE('',#7628,#1712);
#1228=LINE('',#7632,#1713);
#1229=LINE('',#7634,#1714);
#1230=LINE('',#7635,#1715);
#1231=LINE('',#7638,#1716);
#1232=LINE('',#7640,#1717);
#1233=LINE('',#7641,#1718);
#1234=LINE('',#7643,#1719);
#1235=LINE('',#7644,#1720);
#1236=LINE('',#7647,#1721);
#1237=LINE('',#7649,#1722);
#1238=LINE('',#7650,#1723);
#1239=LINE('',#7653,#1724);
#1240=LINE('',#7655,#1725);
#1241=LINE('',#7656,#1726);
#1242=LINE('',#7659,#1727);
#1243=LINE('',#7661,#1728);
#1244=LINE('',#7662,#1729);
#1245=LINE('',#7667,#1730);
#1246=LINE('',#7671,#1731);
#1247=LINE('',#7673,#1732);
#1248=LINE('',#7674,#1733);
#1249=LINE('',#7677,#1734);
#1250=LINE('',#7679,#1735);
#1251=LINE('',#7680,#1736);
#1252=LINE('',#7682,#1737);
#1253=LINE('',#7683,#1738);
#1254=LINE('',#7687,#1739);
#1255=LINE('',#7689,#1740);
#1256=LINE('',#7691,#1741);
#1257=LINE('',#7692,#1742);
#1258=LINE('',#7696,#1743);
#1259=LINE('',#7698,#1744);
#1260=LINE('',#7700,#1745);
#1261=LINE('',#7701,#1746);
#1262=LINE('',#7706,#1747);
#1263=LINE('',#7712,#1748);
#1264=LINE('',#7718,#1749);
#1265=LINE('',#7724,#1750);
#1266=LINE('',#7727,#1751);
#1267=LINE('',#7728,#1752);
#1268=LINE('',#7732,#1753);
#1269=LINE('',#7734,#1754);
#1270=LINE('',#7736,#1755);
#1271=LINE('',#7737,#1756);
#1272=LINE('',#7742,#1757);
#1273=LINE('',#7748,#1758);
#1274=LINE('',#7753,#1759);
#1275=LINE('',#7755,#1760);
#1276=LINE('',#7757,#1761);
#1277=LINE('',#7758,#1762);
#1278=LINE('',#7762,#1763);
#1279=LINE('',#7764,#1764);
#1280=LINE('',#7766,#1765);
#1281=LINE('',#7767,#1766);
#1282=LINE('',#7772,#1767);
#1283=LINE('',#7778,#1768);
#1284=LINE('',#7784,#1769);
#1285=LINE('',#7790,#1770);
#1286=LINE('',#7795,#1771);
#1287=LINE('',#7797,#1772);
#1288=LINE('',#7799,#1773);
#1289=LINE('',#7800,#1774);
#1290=LINE('',#7804,#1775);
#1291=LINE('',#7806,#1776);
#1292=LINE('',#7808,#1777);
#1293=LINE('',#7809,#1778);
#1294=LINE('',#7814,#1779);
#1295=LINE('',#7820,#1780);
#1296=LINE('',#7826,#1781);
#1297=LINE('',#7832,#1782);
#1298=LINE('',#7835,#1783);
#1299=LINE('',#7836,#1784);
#1300=LINE('',#7840,#1785);
#1301=LINE('',#7842,#1786);
#1302=LINE('',#7844,#1787);
#1303=LINE('',#7845,#1788);
#1304=LINE('',#7850,#1789);
#1305=LINE('',#7856,#1790);
#1306=LINE('',#7859,#1791);
#1307=LINE('',#7860,#1792);
#1308=LINE('',#7862,#1793);
#1309=LINE('',#7863,#1794);
#1310=LINE('',#7865,#1795);
#1311=LINE('',#7866,#1796);
#1312=LINE('',#7870,#1797);
#1313=LINE('',#7872,#1798);
#1314=LINE('',#7874,#1799);
#1315=LINE('',#7875,#1800);
#1316=LINE('',#7880,#1801);
#1317=LINE('',#7886,#1802);
#1318=LINE('',#7889,#1803);
#1319=LINE('',#7890,#1804);
#1320=LINE('',#7892,#1805);
#1321=LINE('',#7893,#1806);
#1322=LINE('',#7897,#1807);
#1323=LINE('',#7899,#1808);
#1324=LINE('',#7901,#1809);
#1325=LINE('',#7902,#1810);
#1326=LINE('',#7905,#1811);
#1327=LINE('',#7907,#1812);
#1328=LINE('',#7908,#1813);
#1329=LINE('',#7911,#1814);
#1330=LINE('',#7913,#1815);
#1331=LINE('',#7914,#1816);
#1332=LINE('',#7919,#1817);
#1333=LINE('',#7925,#1818);
#1334=LINE('',#7929,#1819);
#1335=LINE('',#7931,#1820);
#1336=LINE('',#7932,#1821);
#1337=LINE('',#7935,#1822);
#1338=LINE('',#7937,#1823);
#1339=LINE('',#7938,#1824);
#1340=LINE('',#7941,#1825);
#1341=LINE('',#7943,#1826);
#1342=LINE('',#7944,#1827);
#1343=LINE('',#7949,#1828);
#1344=LINE('',#7954,#1829);
#1345=LINE('',#7956,#1830);
#1346=LINE('',#7958,#1831);
#1347=LINE('',#7959,#1832);
#1348=LINE('',#7962,#1833);
#1349=LINE('',#7964,#1834);
#1350=LINE('',#7965,#1835);
#1351=LINE('',#7968,#1836);
#1352=LINE('',#7970,#1837);
#1353=LINE('',#7971,#1838);
#1354=LINE('',#7976,#1839);
#1355=LINE('',#7982,#1840);
#1356=LINE('',#7987,#1841);
#1357=LINE('',#7989,#1842);
#1358=LINE('',#7991,#1843);
#1359=LINE('',#7992,#1844);
#1360=LINE('',#7995,#1845);
#1361=LINE('',#7997,#1846);
#1362=LINE('',#7998,#1847);
#1363=LINE('',#8001,#1848);
#1364=LINE('',#8003,#1849);
#1365=LINE('',#8004,#1850);
#1366=LINE('',#8009,#1851);
#1367=LINE('',#8015,#1852);
#1368=LINE('',#8019,#1853);
#1369=LINE('',#8021,#1854);
#1370=LINE('',#8022,#1855);
#1371=LINE('',#8025,#1856);
#1372=LINE('',#8027,#1857);
#1373=LINE('',#8028,#1858);
#1374=LINE('',#8030,#1859);
#1375=LINE('',#8031,#1860);
#1376=LINE('',#8034,#1861);
#1377=LINE('',#8036,#1862);
#1378=LINE('',#8037,#1863);
#1379=LINE('',#8040,#1864);
#1380=LINE('',#8042,#1865);
#1381=LINE('',#8043,#1866);
#1382=LINE('',#8045,#1867);
#1383=LINE('',#8046,#1868);
#1384=LINE('',#8049,#1869);
#1385=LINE('',#8051,#1870);
#1386=LINE('',#8052,#1871);
#1387=LINE('',#8055,#1872);
#1388=LINE('',#8057,#1873);
#1389=LINE('',#8058,#1874);
#1390=LINE('',#8060,#1875);
#1391=LINE('',#8061,#1876);
#1392=LINE('',#8064,#1877);
#1393=LINE('',#8066,#1878);
#1394=LINE('',#8067,#1879);
#1395=LINE('',#8070,#1880);
#1396=LINE('',#8072,#1881);
#1397=LINE('',#8073,#1882);
#1398=LINE('',#8076,#1883);
#1399=LINE('',#8078,#1884);
#1400=LINE('',#8079,#1885);
#1401=LINE('',#8084,#1886);
#1402=LINE('',#8087,#1887);
#1403=LINE('',#8088,#1888);
#1404=LINE('',#8092,#1889);
#1405=LINE('',#8094,#1890);
#1406=LINE('',#8096,#1891);
#1407=LINE('',#8097,#1892);
#1408=LINE('',#8102,#1893);
#1409=LINE('',#8108,#1894);
#1410=LINE('',#8113,#1895);
#1411=LINE('',#8115,#1896);
#1412=LINE('',#8117,#1897);
#1413=LINE('',#8118,#1898);
#1414=LINE('',#8120,#1899);
#1415=LINE('',#8121,#1900);
#1416=LINE('',#8126,#1901);
#1417=LINE('',#8132,#1902);
#1418=LINE('',#8135,#1903);
#1419=LINE('',#8136,#1904);
#1420=LINE('',#8138,#1905);
#1421=LINE('',#8139,#1906);
#1422=LINE('',#8143,#1907);
#1423=LINE('',#8145,#1908);
#1424=LINE('',#8147,#1909);
#1425=LINE('',#8148,#1910);
#1426=LINE('',#8151,#1911);
#1427=LINE('',#8153,#1912);
#1428=LINE('',#8154,#1913);
#1429=LINE('',#8157,#1914);
#1430=LINE('',#8159,#1915);
#1431=LINE('',#8160,#1916);
#1432=LINE('',#8165,#1917);
#1433=LINE('',#8171,#1918);
#1434=LINE('',#8175,#1919);
#1435=LINE('',#8177,#1920);
#1436=LINE('',#8178,#1921);
#1437=LINE('',#8181,#1922);
#1438=LINE('',#8183,#1923);
#1439=LINE('',#8184,#1924);
#1440=LINE('',#8187,#1925);
#1441=LINE('',#8189,#1926);
#1442=LINE('',#8190,#1927);
#1443=LINE('',#8195,#1928);
#1444=LINE('',#8200,#1929);
#1445=LINE('',#8202,#1930);
#1446=LINE('',#8204,#1931);
#1447=LINE('',#8205,#1932);
#1448=LINE('',#8208,#1933);
#1449=LINE('',#8210,#1934);
#1450=LINE('',#8211,#1935);
#1451=LINE('',#8214,#1936);
#1452=LINE('',#8216,#1937);
#1453=LINE('',#8217,#1938);
#1454=LINE('',#8222,#1939);
#1455=LINE('',#8228,#1940);
#1456=LINE('',#8232,#1941);
#1457=LINE('',#8234,#1942);
#1458=LINE('',#8235,#1943);
#1459=LINE('',#8238,#1944);
#1460=LINE('',#8240,#1945);
#1461=LINE('',#8241,#1946);
#1462=LINE('',#8244,#1947);
#1463=LINE('',#8246,#1948);
#1464=LINE('',#8247,#1949);
#1465=LINE('',#8252,#1950);
#1466=LINE('',#8256,#1951);
#1467=LINE('',#8258,#1952);
#1468=LINE('',#8259,#1953);
#1469=LINE('',#8262,#1954);
#1470=LINE('',#8264,#1955);
#1471=LINE('',#8265,#1956);
#1472=LINE('',#8268,#1957);
#1473=LINE('',#8270,#1958);
#1474=LINE('',#8271,#1959);
#1475=LINE('',#8276,#1960);
#1476=LINE('',#8280,#1961);
#1477=LINE('',#8282,#1962);
#1478=LINE('',#8283,#1963);
#1479=LINE('',#8286,#1964);
#1480=LINE('',#8288,#1965);
#1481=LINE('',#8289,#1966);
#1482=LINE('',#8291,#1967);
#1483=LINE('',#8292,#1968);
#1484=LINE('',#8295,#1969);
#1485=LINE('',#8297,#1970);
#1486=LINE('',#8298,#1971);
#1487=LINE('',#8301,#1972);
#1488=LINE('',#8303,#1973);
#1489=LINE('',#8304,#1974);
#1490=LINE('',#8306,#1975);
#1491=LINE('',#8307,#1976);
#1492=LINE('',#8310,#1977);
#1493=LINE('',#8312,#1978);
#1494=LINE('',#8313,#1979);
#1495=LINE('',#8316,#1980);
#1496=LINE('',#8318,#1981);
#1497=LINE('',#8319,#1982);
#1498=LINE('',#8321,#1983);
#1499=LINE('',#8322,#1984);
#1500=LINE('',#8324,#1985);
#1501=LINE('',#8325,#1986);
#1502=LINE('',#8327,#1987);
#1503=LINE('',#8328,#1988);
#1504=LINE('',#8333,#1989);
#1569=VECTOR('',#5728,10.);
#1570=VECTOR('',#5729,10.);
#1571=VECTOR('',#5730,10.);
#1572=VECTOR('',#5731,10.);
#1573=VECTOR('',#5734,10.);
#1574=VECTOR('',#5735,10.);
#1575=VECTOR('',#5736,10.);
#1576=VECTOR('',#5739,10.);
#1577=VECTOR('',#5740,10.);
#1578=VECTOR('',#5741,10.);
#1579=VECTOR('',#5746,10.);
#1580=VECTOR('',#5753,10.);
#1581=VECTOR('',#5758,10.);
#1582=VECTOR('',#5759,10.);
#1583=VECTOR('',#5760,10.);
#1584=VECTOR('',#5761,10.);
#1585=VECTOR('',#5764,10.);
#1586=VECTOR('',#5765,10.);
#1587=VECTOR('',#5766,10.);
#1588=VECTOR('',#5769,10.);
#1589=VECTOR('',#5770,10.);
#1590=VECTOR('',#5771,10.);
#1591=VECTOR('',#5776,10.);
#1592=VECTOR('',#5783,10.);
#1593=VECTOR('',#5788,10.);
#1594=VECTOR('',#5789,10.);
#1595=VECTOR('',#5790,10.);
#1596=VECTOR('',#5793,10.);
#1597=VECTOR('',#5794,10.);
#1598=VECTOR('',#5795,10.);
#1599=VECTOR('',#5798,10.);
#1600=VECTOR('',#5799,10.);
#1601=VECTOR('',#5800,10.);
#1602=VECTOR('',#5805,10.);
#1603=VECTOR('',#5810,10.);
#1604=VECTOR('',#5811,10.);
#1605=VECTOR('',#5812,10.);
#1606=VECTOR('',#5813,10.);
#1607=VECTOR('',#5816,10.);
#1608=VECTOR('',#5817,10.);
#1609=VECTOR('',#5818,10.);
#1610=VECTOR('',#5821,10.);
#1611=VECTOR('',#5822,10.);
#1612=VECTOR('',#5823,10.);
#1613=VECTOR('',#5828,10.);
#1614=VECTOR('',#5835,10.);
#1615=VECTOR('',#5840,10.);
#1616=VECTOR('',#5841,10.);
#1617=VECTOR('',#5842,10.);
#1618=VECTOR('',#5845,10.);
#1619=VECTOR('',#5846,10.);
#1620=VECTOR('',#5847,10.);
#1621=VECTOR('',#5850,10.);
#1622=VECTOR('',#5851,10.);
#1623=VECTOR('',#5854,10.);
#1624=VECTOR('',#5855,10.);
#1625=VECTOR('',#5856,10.);
#1626=VECTOR('',#5859,10.);
#1627=VECTOR('',#5860,10.);
#1628=VECTOR('',#5861,10.);
#1629=VECTOR('',#5864,10.);
#1630=VECTOR('',#5865,10.);
#1631=VECTOR('',#5866,10.);
#1632=VECTOR('',#5871,10.);
#1633=VECTOR('',#5876,10.);
#1634=VECTOR('',#5877,10.);
#1635=VECTOR('',#5878,10.);
#1636=VECTOR('',#5879,10.);
#1637=VECTOR('',#5882,9.99999999999999);
#1638=VECTOR('',#5883,10.);
#1639=VECTOR('',#5884,10.);
#1640=VECTOR('',#5887,10.);
#1641=VECTOR('',#5888,10.);
#1642=VECTOR('',#5893,10.);
#1643=VECTOR('',#5898,10.);
#1644=VECTOR('',#5899,9.99999999999998);
#1645=VECTOR('',#5900,10.);
#1646=VECTOR('',#5903,10.);
#1647=VECTOR('',#5904,10.);
#1648=VECTOR('',#5905,10.);
#1649=VECTOR('',#5908,10.);
#1650=VECTOR('',#5909,10.);
#1651=VECTOR('',#5912,10.);
#1652=VECTOR('',#5913,10.);
#1653=VECTOR('',#5914,10.);
#1654=VECTOR('',#5915,10.);
#1655=VECTOR('',#5918,10.);
#1656=VECTOR('',#5919,10.);
#1657=VECTOR('',#5920,10.);
#1658=VECTOR('',#5921,10.);
#1659=VECTOR('',#5926,10.);
#1660=VECTOR('',#5933,10.);
#1661=VECTOR('',#5940,10.);
#1662=VECTOR('',#5947,10.);
#1663=VECTOR('',#5952,10.);
#1664=VECTOR('',#5953,10.);
#1665=VECTOR('',#5956,10.);
#1666=VECTOR('',#5957,10.);
#1667=VECTOR('',#5958,10.);
#1668=VECTOR('',#5959,10.);
#1669=VECTOR('',#5964,10.);
#1670=VECTOR('',#5971,10.);
#1671=VECTOR('',#5976,10.);
#1672=VECTOR('',#5977,10.);
#1673=VECTOR('',#5978,10.);
#1674=VECTOR('',#5979,10.);
#1675=VECTOR('',#5982,10.);
#1676=VECTOR('',#5983,10.);
#1677=VECTOR('',#5988,10.);
#1678=VECTOR('',#5995,10.);
#1679=VECTOR('',#6000,10.);
#1680=VECTOR('',#6001,10.);
#1681=VECTOR('',#6002,10.);
#1682=VECTOR('',#6003,10.);
#1683=VECTOR('',#6006,10.);
#1684=VECTOR('',#6007,9.99999999999999);
#1685=VECTOR('',#6008,10.);
#1686=VECTOR('',#6011,10.);
#1687=VECTOR('',#6012,10.);
#1688=VECTOR('',#6013,10.);
#1689=VECTOR('',#6018,10.);
#1690=VECTOR('',#6025,10.);
#1691=VECTOR('',#6030,9.99999999999998);
#1692=VECTOR('',#6031,10.);
#1693=VECTOR('',#6032,9.99999999999998);
#1694=VECTOR('',#6033,10.);
#1695=VECTOR('',#6036,10.);
#1696=VECTOR('',#6037,10.);
#1697=VECTOR('',#6038,10.);
#1698=VECTOR('',#6041,10.);
#1699=VECTOR('',#6042,10.);
#1700=VECTOR('',#6043,10.);
#1701=VECTOR('',#6048,10.);
#1702=VECTOR('',#6055,10.);
#1703=VECTOR('',#6060,10.);
#1704=VECTOR('',#6061,10.);
#1705=VECTOR('',#6062,10.);
#1706=VECTOR('',#6065,10.);
#1707=VECTOR('',#6066,10.);
#1708=VECTOR('',#6067,10.);
#1709=VECTOR('',#6070,10.);
#1710=VECTOR('',#6071,10.);
#1711=VECTOR('',#6072,10.);
#1712=VECTOR('',#6077,10.);
#1713=VECTOR('',#6082,10.);
#1714=VECTOR('',#6083,10.);
#1715=VECTOR('',#6084,10.);
#1716=VECTOR('',#6087,10.);
#1717=VECTOR('',#6088,10.);
#1718=VECTOR('',#6089,10.);
#1719=VECTOR('',#6092,10.);
#1720=VECTOR('',#6093,10.);
#1721=VECTOR('',#6096,10.);
#1722=VECTOR('',#6097,10.);
#1723=VECTOR('',#6098,10.);
#1724=VECTOR('',#6101,10.);
#1725=VECTOR('',#6102,10.);
#1726=VECTOR('',#6103,10.);
#1727=VECTOR('',#6106,10.);
#1728=VECTOR('',#6107,10.);
#1729=VECTOR('',#6108,10.);
#1730=VECTOR('',#6113,10.);
#1731=VECTOR('',#6118,10.);
#1732=VECTOR('',#6119,10.);
#1733=VECTOR('',#6120,10.);
#1734=VECTOR('',#6123,10.);
#1735=VECTOR('',#6124,10.);
#1736=VECTOR('',#6125,10.);
#1737=VECTOR('',#6128,10.);
#1738=VECTOR('',#6129,10.);
#1739=VECTOR('',#6132,9.99999999999998);
#1740=VECTOR('',#6133,10.);
#1741=VECTOR('',#6134,9.99999999999998);
#1742=VECTOR('',#6135,10.);
#1743=VECTOR('',#6138,9.99999999999998);
#1744=VECTOR('',#6139,10.);
#1745=VECTOR('',#6140,9.99999999999998);
#1746=VECTOR('',#6141,10.);
#1747=VECTOR('',#6146,10.);
#1748=VECTOR('',#6153,10.);
#1749=VECTOR('',#6160,10.);
#1750=VECTOR('',#6167,10.);
#1751=VECTOR('',#6172,9.99999999999999);
#1752=VECTOR('',#6173,9.99999999999999);
#1753=VECTOR('',#6176,9.99999999999999);
#1754=VECTOR('',#6177,10.);
#1755=VECTOR('',#6178,9.99999999999999);
#1756=VECTOR('',#6179,10.);
#1757=VECTOR('',#6184,10.);
#1758=VECTOR('',#6191,10.);
#1759=VECTOR('',#6196,10.);
#1760=VECTOR('',#6197,10.);
#1761=VECTOR('',#6198,10.);
#1762=VECTOR('',#6199,10.);
#1763=VECTOR('',#6202,10.);
#1764=VECTOR('',#6203,10.);
#1765=VECTOR('',#6204,10.);
#1766=VECTOR('',#6205,10.);
#1767=VECTOR('',#6210,10.);
#1768=VECTOR('',#6217,10.);
#1769=VECTOR('',#6224,10.);
#1770=VECTOR('',#6231,10.);
#1771=VECTOR('',#6236,10.);
#1772=VECTOR('',#6237,10.);
#1773=VECTOR('',#6238,10.);
#1774=VECTOR('',#6239,10.);
#1775=VECTOR('',#6242,10.);
#1776=VECTOR('',#6243,10.);
#1777=VECTOR('',#6244,10.);
#1778=VECTOR('',#6245,10.);
#1779=VECTOR('',#6250,10.);
#1780=VECTOR('',#6257,10.);
#1781=VECTOR('',#6264,10.);
#1782=VECTOR('',#6271,10.);
#1783=VECTOR('',#6276,10.);
#1784=VECTOR('',#6277,10.);
#1785=VECTOR('',#6280,10.);
#1786=VECTOR('',#6281,10.);
#1787=VECTOR('',#6282,10.);
#1788=VECTOR('',#6283,10.);
#1789=VECTOR('',#6288,10.);
#1790=VECTOR('',#6295,10.);
#1791=VECTOR('',#6300,10.);
#1792=VECTOR('',#6301,10.);
#1793=VECTOR('',#6304,10.);
#1794=VECTOR('',#6305,10.);
#1795=VECTOR('',#6308,9.99999999999998);
#1796=VECTOR('',#6309,9.99999999999998);
#1797=VECTOR('',#6312,9.99999999999998);
#1798=VECTOR('',#6313,10.);
#1799=VECTOR('',#6314,9.99999999999998);
#1800=VECTOR('',#6315,10.);
#1801=VECTOR('',#6320,10.);
#1802=VECTOR('',#6327,10.);
#1803=VECTOR('',#6332,10.);
#1804=VECTOR('',#6333,10.);
#1805=VECTOR('',#6336,10.);
#1806=VECTOR('',#6337,10.);
#1807=VECTOR('',#6340,9.99999999999998);
#1808=VECTOR('',#6341,10.);
#1809=VECTOR('',#6342,9.99999999999998);
#1810=VECTOR('',#6343,10.);
#1811=VECTOR('',#6346,10.);
#1812=VECTOR('',#6347,10.);
#1813=VECTOR('',#6348,10.);
#1814=VECTOR('',#6351,10.);
#1815=VECTOR('',#6352,10.);
#1816=VECTOR('',#6353,10.);
#1817=VECTOR('',#6358,10.);
#1818=VECTOR('',#6365,10.);
#1819=VECTOR('',#6370,10.);
#1820=VECTOR('',#6371,10.);
#1821=VECTOR('',#6372,10.);
#1822=VECTOR('',#6375,10.);
#1823=VECTOR('',#6376,10.);
#1824=VECTOR('',#6377,10.);
#1825=VECTOR('',#6380,10.);
#1826=VECTOR('',#6381,10.);
#1827=VECTOR('',#6382,10.);
#1828=VECTOR('',#6387,10.);
#1829=VECTOR('',#6392,10.);
#1830=VECTOR('',#6393,10.);
#1831=VECTOR('',#6394,10.);
#1832=VECTOR('',#6395,10.);
#1833=VECTOR('',#6398,10.);
#1834=VECTOR('',#6399,9.99999999999999);
#1835=VECTOR('',#6400,10.);
#1836=VECTOR('',#6403,10.);
#1837=VECTOR('',#6404,10.);
#1838=VECTOR('',#6405,10.);
#1839=VECTOR('',#6410,10.);
#1840=VECTOR('',#6417,10.);
#1841=VECTOR('',#6422,10.);
#1842=VECTOR('',#6423,10.);
#1843=VECTOR('',#6424,10.);
#1844=VECTOR('',#6425,10.);
#1845=VECTOR('',#6428,10.);
#1846=VECTOR('',#6429,10.);
#1847=VECTOR('',#6430,10.);
#1848=VECTOR('',#6433,10.);
#1849=VECTOR('',#6434,10.);
#1850=VECTOR('',#6435,10.);
#1851=VECTOR('',#6440,10.);
#1852=VECTOR('',#6447,10.);
#1853=VECTOR('',#6452,10.);
#1854=VECTOR('',#6453,10.);
#1855=VECTOR('',#6454,10.);
#1856=VECTOR('',#6457,10.);
#1857=VECTOR('',#6458,10.);
#1858=VECTOR('',#6459,10.);
#1859=VECTOR('',#6462,10.);
#1860=VECTOR('',#6463,10.);
#1861=VECTOR('',#6466,10.);
#1862=VECTOR('',#6467,10.);
#1863=VECTOR('',#6468,10.);
#1864=VECTOR('',#6471,10.);
#1865=VECTOR('',#6472,10.);
#1866=VECTOR('',#6473,10.);
#1867=VECTOR('',#6476,10.);
#1868=VECTOR('',#6477,10.);
#1869=VECTOR('',#6480,10.);
#1870=VECTOR('',#6481,10.);
#1871=VECTOR('',#6482,10.);
#1872=VECTOR('',#6485,10.);
#1873=VECTOR('',#6486,9.99999999999999);
#1874=VECTOR('',#6487,10.);
#1875=VECTOR('',#6490,10.);
#1876=VECTOR('',#6491,10.);
#1877=VECTOR('',#6494,10.);
#1878=VECTOR('',#6495,10.);
#1879=VECTOR('',#6496,10.);
#1880=VECTOR('',#6499,10.);
#1881=VECTOR('',#6500,10.);
#1882=VECTOR('',#6501,10.);
#1883=VECTOR('',#6504,10.);
#1884=VECTOR('',#6505,10.);
#1885=VECTOR('',#6506,10.);
#1886=VECTOR('',#6511,10.);
#1887=VECTOR('',#6516,9.99999999999999);
#1888=VECTOR('',#6517,9.99999999999999);
#1889=VECTOR('',#6520,9.99999999999999);
#1890=VECTOR('',#6521,10.);
#1891=VECTOR('',#6522,9.99999999999999);
#1892=VECTOR('',#6523,10.);
#1893=VECTOR('',#6528,10.);
#1894=VECTOR('',#6535,10.);
#1895=VECTOR('',#6540,10.);
#1896=VECTOR('',#6541,10.);
#1897=VECTOR('',#6542,10.);
#1898=VECTOR('',#6543,10.);
#1899=VECTOR('',#6546,10.);
#1900=VECTOR('',#6547,10.);
#1901=VECTOR('',#6552,10.);
#1902=VECTOR('',#6559,10.);
#1903=VECTOR('',#6564,10.);
#1904=VECTOR('',#6565,10.);
#1905=VECTOR('',#6568,10.);
#1906=VECTOR('',#6569,10.);
#1907=VECTOR('',#6572,10.);
#1908=VECTOR('',#6573,10.);
#1909=VECTOR('',#6574,10.);
#1910=VECTOR('',#6575,10.);
#1911=VECTOR('',#6578,10.);
#1912=VECTOR('',#6579,10.);
#1913=VECTOR('',#6580,10.);
#1914=VECTOR('',#6583,10.);
#1915=VECTOR('',#6584,10.);
#1916=VECTOR('',#6585,10.);
#1917=VECTOR('',#6590,10.);
#1918=VECTOR('',#6597,10.);
#1919=VECTOR('',#6602,10.);
#1920=VECTOR('',#6603,10.);
#1921=VECTOR('',#6604,10.);
#1922=VECTOR('',#6607,10.);
#1923=VECTOR('',#6608,10.);
#1924=VECTOR('',#6609,10.);
#1925=VECTOR('',#6612,10.);
#1926=VECTOR('',#6613,10.);
#1927=VECTOR('',#6614,10.);
#1928=VECTOR('',#6619,10.);
#1929=VECTOR('',#6624,10.);
#1930=VECTOR('',#6625,10.);
#1931=VECTOR('',#6626,10.);
#1932=VECTOR('',#6627,10.);
#1933=VECTOR('',#6630,10.);
#1934=VECTOR('',#6631,10.);
#1935=VECTOR('',#6632,10.);
#1936=VECTOR('',#6635,10.);
#1937=VECTOR('',#6636,10.);
#1938=VECTOR('',#6637,10.);
#1939=VECTOR('',#6642,10.);
#1940=VECTOR('',#6649,10.);
#1941=VECTOR('',#6654,10.);
#1942=VECTOR('',#6655,10.);
#1943=VECTOR('',#6656,10.);
#1944=VECTOR('',#6659,10.);
#1945=VECTOR('',#6660,10.);
#1946=VECTOR('',#6661,10.);
#1947=VECTOR('',#6664,10.);
#1948=VECTOR('',#6665,10.);
#1949=VECTOR('',#6666,10.);
#1950=VECTOR('',#6671,10.);
#1951=VECTOR('',#6676,10.);
#1952=VECTOR('',#6677,10.);
#1953=VECTOR('',#6678,10.);
#1954=VECTOR('',#6681,10.);
#1955=VECTOR('',#6682,10.);
#1956=VECTOR('',#6683,10.);
#1957=VECTOR('',#6686,10.);
#1958=VECTOR('',#6687,10.);
#1959=VECTOR('',#6688,10.);
#1960=VECTOR('',#6693,10.);
#1961=VECTOR('',#6698,10.);
#1962=VECTOR('',#6699,10.);
#1963=VECTOR('',#6700,10.);
#1964=VECTOR('',#6703,10.);
#1965=VECTOR('',#6704,10.);
#1966=VECTOR('',#6705,10.);
#1967=VECTOR('',#6708,10.);
#1968=VECTOR('',#6709,10.);
#1969=VECTOR('',#6712,10.);
#1970=VECTOR('',#6713,10.);
#1971=VECTOR('',#6714,10.);
#1972=VECTOR('',#6717,9.99999999999999);
#1973=VECTOR('',#6718,9.99999999999999);
#1974=VECTOR('',#6719,10.);
#1975=VECTOR('',#6722,10.);
#1976=VECTOR('',#6723,10.);
#1977=VECTOR('',#6726,10.);
#1978=VECTOR('',#6727,10.);
#1979=VECTOR('',#6728,10.);
#1980=VECTOR('',#6731,10.);
#1981=VECTOR('',#6732,10.);
#1982=VECTOR('',#6733,10.);
#1983=VECTOR('',#6736,10.);
#1984=VECTOR('',#6737,10.);
#1985=VECTOR('',#6740,10.);
#1986=VECTOR('',#6741,10.);
#1987=VECTOR('',#6744,10.);
#1988=VECTOR('',#6745,10.);
#1989=VECTOR('',#6750,1.99137169252308);
#2054=VERTEX_POINT('',#7250);
#2055=VERTEX_POINT('',#7251);
#2056=VERTEX_POINT('',#7253);
#2057=VERTEX_POINT('',#7255);
#2058=VERTEX_POINT('',#7259);
#2059=VERTEX_POINT('',#7261);
#2060=VERTEX_POINT('',#7265);
#2061=VERTEX_POINT('',#7267);
#2062=VERTEX_POINT('',#7271);
#2063=VERTEX_POINT('',#7273);
#2064=VERTEX_POINT('',#7277);
#2065=VERTEX_POINT('',#7279);
#2066=VERTEX_POINT('',#7283);
#2067=VERTEX_POINT('',#7284);
#2068=VERTEX_POINT('',#7286);
#2069=VERTEX_POINT('',#7288);
#2070=VERTEX_POINT('',#7292);
#2071=VERTEX_POINT('',#7294);
#2072=VERTEX_POINT('',#7298);
#2073=VERTEX_POINT('',#7300);
#2074=VERTEX_POINT('',#7304);
#2075=VERTEX_POINT('',#7306);
#2076=VERTEX_POINT('',#7310);
#2077=VERTEX_POINT('',#7312);
#2078=VERTEX_POINT('',#7316);
#2079=VERTEX_POINT('',#7318);
#2080=VERTEX_POINT('',#7322);
#2081=VERTEX_POINT('',#7324);
#2082=VERTEX_POINT('',#7328);
#2083=VERTEX_POINT('',#7330);
#2084=VERTEX_POINT('',#7334);
#2085=VERTEX_POINT('',#7336);
#2086=VERTEX_POINT('',#7340);
#2087=VERTEX_POINT('',#7341);
#2088=VERTEX_POINT('',#7343);
#2089=VERTEX_POINT('',#7345);
#2090=VERTEX_POINT('',#7349);
#2091=VERTEX_POINT('',#7351);
#2092=VERTEX_POINT('',#7355);
#2093=VERTEX_POINT('',#7357);
#2094=VERTEX_POINT('',#7361);
#2095=VERTEX_POINT('',#7363);
#2096=VERTEX_POINT('',#7367);
#2097=VERTEX_POINT('',#7369);
#2098=VERTEX_POINT('',#7373);
#2099=VERTEX_POINT('',#7375);
#2100=VERTEX_POINT('',#7379);
#2101=VERTEX_POINT('',#7381);
#2102=VERTEX_POINT('',#7388);
#2103=VERTEX_POINT('',#7390);
#2104=VERTEX_POINT('',#7394);
#2105=VERTEX_POINT('',#7396);
#2106=VERTEX_POINT('',#7400);
#2107=VERTEX_POINT('',#7402);
#2108=VERTEX_POINT('',#7406);
#2109=VERTEX_POINT('',#7408);
#2110=VERTEX_POINT('',#7412);
#2111=VERTEX_POINT('',#7413);
#2112=VERTEX_POINT('',#7415);
#2113=VERTEX_POINT('',#7417);
#2114=VERTEX_POINT('',#7421);
#2115=VERTEX_POINT('',#7423);
#2116=VERTEX_POINT('',#7430);
#2117=VERTEX_POINT('',#7432);
#2118=VERTEX_POINT('',#7436);
#2119=VERTEX_POINT('',#7438);
#2120=VERTEX_POINT('',#7442);
#2121=VERTEX_POINT('',#7444);
#2122=VERTEX_POINT('',#7451);
#2123=VERTEX_POINT('',#7452);
#2124=VERTEX_POINT('',#7454);
#2125=VERTEX_POINT('',#7456);
#2126=VERTEX_POINT('',#7460);
#2127=VERTEX_POINT('',#7461);
#2128=VERTEX_POINT('',#7463);
#2129=VERTEX_POINT('',#7465);
#2130=VERTEX_POINT('',#7469);
#2131=VERTEX_POINT('',#7471);
#2132=VERTEX_POINT('',#7475);
#2133=VERTEX_POINT('',#7477);
#2134=VERTEX_POINT('',#7481);
#2135=VERTEX_POINT('',#7483);
#2136=VERTEX_POINT('',#7487);
#2137=VERTEX_POINT('',#7489);
#2138=VERTEX_POINT('',#7496);
#2139=VERTEX_POINT('',#7497);
#2140=VERTEX_POINT('',#7499);
#2141=VERTEX_POINT('',#7501);
#2142=VERTEX_POINT('',#7505);
#2143=VERTEX_POINT('',#7507);
#2144=VERTEX_POINT('',#7511);
#2145=VERTEX_POINT('',#7513);
#2146=VERTEX_POINT('',#7517);
#2147=VERTEX_POINT('',#7518);
#2148=VERTEX_POINT('',#7520);
#2149=VERTEX_POINT('',#7522);
#2150=VERTEX_POINT('',#7529);
#2151=VERTEX_POINT('',#7531);
#2152=VERTEX_POINT('',#7535);
#2153=VERTEX_POINT('',#7537);
#2154=VERTEX_POINT('',#7541);
#2155=VERTEX_POINT('',#7542);
#2156=VERTEX_POINT('',#7544);
#2157=VERTEX_POINT('',#7546);
#2158=VERTEX_POINT('',#7550);
#2159=VERTEX_POINT('',#7552);
#2160=VERTEX_POINT('',#7556);
#2161=VERTEX_POINT('',#7558);
#2162=VERTEX_POINT('',#7562);
#2163=VERTEX_POINT('',#7564);
#2164=VERTEX_POINT('',#7568);
#2165=VERTEX_POINT('',#7570);
#2166=VERTEX_POINT('',#7574);
#2167=VERTEX_POINT('',#7575);
#2168=VERTEX_POINT('',#7577);
#2169=VERTEX_POINT('',#7579);
#2170=VERTEX_POINT('',#7583);
#2171=VERTEX_POINT('',#7585);
#2172=VERTEX_POINT('',#7589);
#2173=VERTEX_POINT('',#7591);
#2174=VERTEX_POINT('',#7595);
#2175=VERTEX_POINT('',#7597);
#2176=VERTEX_POINT('',#7601);
#2177=VERTEX_POINT('',#7603);
#2178=VERTEX_POINT('',#7607);
#2179=VERTEX_POINT('',#7609);
#2180=VERTEX_POINT('',#7613);
#2181=VERTEX_POINT('',#7615);
#2182=VERTEX_POINT('',#7619);
#2183=VERTEX_POINT('',#7621);
#2184=VERTEX_POINT('',#7625);
#2185=VERTEX_POINT('',#7627);
#2186=VERTEX_POINT('',#7631);
#2187=VERTEX_POINT('',#7633);
#2188=VERTEX_POINT('',#7637);
#2189=VERTEX_POINT('',#7639);
#2190=VERTEX_POINT('',#7646);
#2191=VERTEX_POINT('',#7648);
#2192=VERTEX_POINT('',#7652);
#2193=VERTEX_POINT('',#7654);
#2194=VERTEX_POINT('',#7658);
#2195=VERTEX_POINT('',#7660);
#2196=VERTEX_POINT('',#7664);
#2197=VERTEX_POINT('',#7666);
#2198=VERTEX_POINT('',#7670);
#2199=VERTEX_POINT('',#7672);
#2200=VERTEX_POINT('',#7676);
#2201=VERTEX_POINT('',#7678);
#2202=VERTEX_POINT('',#7685);
#2203=VERTEX_POINT('',#7686);
#2204=VERTEX_POINT('',#7688);
#2205=VERTEX_POINT('',#7690);
#2206=VERTEX_POINT('',#7694);
#2207=VERTEX_POINT('',#7695);
#2208=VERTEX_POINT('',#7697);
#2209=VERTEX_POINT('',#7699);
#2210=VERTEX_POINT('',#7703);
#2211=VERTEX_POINT('',#7705);
#2212=VERTEX_POINT('',#7709);
#2213=VERTEX_POINT('',#7711);
#2214=VERTEX_POINT('',#7715);
#2215=VERTEX_POINT('',#7717);
#2216=VERTEX_POINT('',#7721);
#2217=VERTEX_POINT('',#7723);
#2218=VERTEX_POINT('',#7730);
#2219=VERTEX_POINT('',#7731);
#2220=VERTEX_POINT('',#7733);
#2221=VERTEX_POINT('',#7735);
#2222=VERTEX_POINT('',#7739);
#2223=VERTEX_POINT('',#7741);
#2224=VERTEX_POINT('',#7745);
#2225=VERTEX_POINT('',#7747);
#2226=VERTEX_POINT('',#7751);
#2227=VERTEX_POINT('',#7752);
#2228=VERTEX_POINT('',#7754);
#2229=VERTEX_POINT('',#7756);
#2230=VERTEX_POINT('',#7760);
#2231=VERTEX_POINT('',#7761);
#2232=VERTEX_POINT('',#7763);
#2233=VERTEX_POINT('',#7765);
#2234=VERTEX_POINT('',#7769);
#2235=VERTEX_POINT('',#7771);
#2236=VERTEX_POINT('',#7775);
#2237=VERTEX_POINT('',#7777);
#2238=VERTEX_POINT('',#7781);
#2239=VERTEX_POINT('',#7783);
#2240=VERTEX_POINT('',#7787);
#2241=VERTEX_POINT('',#7789);
#2242=VERTEX_POINT('',#7793);
#2243=VERTEX_POINT('',#7794);
#2244=VERTEX_POINT('',#7796);
#2245=VERTEX_POINT('',#7798);
#2246=VERTEX_POINT('',#7802);
#2247=VERTEX_POINT('',#7803);
#2248=VERTEX_POINT('',#7805);
#2249=VERTEX_POINT('',#7807);
#2250=VERTEX_POINT('',#7811);
#2251=VERTEX_POINT('',#7813);
#2252=VERTEX_POINT('',#7817);
#2253=VERTEX_POINT('',#7819);
#2254=VERTEX_POINT('',#7823);
#2255=VERTEX_POINT('',#7825);
#2256=VERTEX_POINT('',#7829);
#2257=VERTEX_POINT('',#7831);
#2258=VERTEX_POINT('',#7838);
#2259=VERTEX_POINT('',#7839);
#2260=VERTEX_POINT('',#7841);
#2261=VERTEX_POINT('',#7843);
#2262=VERTEX_POINT('',#7847);
#2263=VERTEX_POINT('',#7849);
#2264=VERTEX_POINT('',#7853);
#2265=VERTEX_POINT('',#7855);
#2266=VERTEX_POINT('',#7868);
#2267=VERTEX_POINT('',#7869);
#2268=VERTEX_POINT('',#7871);
#2269=VERTEX_POINT('',#7873);
#2270=VERTEX_POINT('',#7877);
#2271=VERTEX_POINT('',#7879);
#2272=VERTEX_POINT('',#7883);
#2273=VERTEX_POINT('',#7885);
#2274=VERTEX_POINT('',#7895);
#2275=VERTEX_POINT('',#7896);
#2276=VERTEX_POINT('',#7898);
#2277=VERTEX_POINT('',#7900);
#2278=VERTEX_POINT('',#7904);
#2279=VERTEX_POINT('',#7906);
#2280=VERTEX_POINT('',#7910);
#2281=VERTEX_POINT('',#7912);
#2282=VERTEX_POINT('',#7916);
#2283=VERTEX_POINT('',#7918);
#2284=VERTEX_POINT('',#7922);
#2285=VERTEX_POINT('',#7924);
#2286=VERTEX_POINT('',#7928);
#2287=VERTEX_POINT('',#7930);
#2288=VERTEX_POINT('',#7934);
#2289=VERTEX_POINT('',#7936);
#2290=VERTEX_POINT('',#7940);
#2291=VERTEX_POINT('',#7942);
#2292=VERTEX_POINT('',#7946);
#2293=VERTEX_POINT('',#7948);
#2294=VERTEX_POINT('',#7952);
#2295=VERTEX_POINT('',#7953);
#2296=VERTEX_POINT('',#7955);
#2297=VERTEX_POINT('',#7957);
#2298=VERTEX_POINT('',#7961);
#2299=VERTEX_POINT('',#7963);
#2300=VERTEX_POINT('',#7967);
#2301=VERTEX_POINT('',#7969);
#2302=VERTEX_POINT('',#7973);
#2303=VERTEX_POINT('',#7975);
#2304=VERTEX_POINT('',#7979);
#2305=VERTEX_POINT('',#7981);
#2306=VERTEX_POINT('',#7985);
#2307=VERTEX_POINT('',#7986);
#2308=VERTEX_POINT('',#7988);
#2309=VERTEX_POINT('',#7990);
#2310=VERTEX_POINT('',#7994);
#2311=VERTEX_POINT('',#7996);
#2312=VERTEX_POINT('',#8000);
#2313=VERTEX_POINT('',#8002);
#2314=VERTEX_POINT('',#8006);
#2315=VERTEX_POINT('',#8008);
#2316=VERTEX_POINT('',#8012);
#2317=VERTEX_POINT('',#8014);
#2318=VERTEX_POINT('',#8018);
#2319=VERTEX_POINT('',#8020);
#2320=VERTEX_POINT('',#8024);
#2321=VERTEX_POINT('',#8026);
#2322=VERTEX_POINT('',#8033);
#2323=VERTEX_POINT('',#8035);
#2324=VERTEX_POINT('',#8039);
#2325=VERTEX_POINT('',#8041);
#2326=VERTEX_POINT('',#8048);
#2327=VERTEX_POINT('',#8050);
#2328=VERTEX_POINT('',#8054);
#2329=VERTEX_POINT('',#8056);
#2330=VERTEX_POINT('',#8063);
#2331=VERTEX_POINT('',#8065);
#2332=VERTEX_POINT('',#8069);
#2333=VERTEX_POINT('',#8071);
#2334=VERTEX_POINT('',#8075);
#2335=VERTEX_POINT('',#8077);
#2336=VERTEX_POINT('',#8081);
#2337=VERTEX_POINT('',#8083);
#2338=VERTEX_POINT('',#8090);
#2339=VERTEX_POINT('',#8091);
#2340=VERTEX_POINT('',#8093);
#2341=VERTEX_POINT('',#8095);
#2342=VERTEX_POINT('',#8099);
#2343=VERTEX_POINT('',#8101);
#2344=VERTEX_POINT('',#8105);
#2345=VERTEX_POINT('',#8107);
#2346=VERTEX_POINT('',#8111);
#2347=VERTEX_POINT('',#8112);
#2348=VERTEX_POINT('',#8114);
#2349=VERTEX_POINT('',#8116);
#2350=VERTEX_POINT('',#8123);
#2351=VERTEX_POINT('',#8125);
#2352=VERTEX_POINT('',#8129);
#2353=VERTEX_POINT('',#8131);
#2354=VERTEX_POINT('',#8141);
#2355=VERTEX_POINT('',#8142);
#2356=VERTEX_POINT('',#8144);
#2357=VERTEX_POINT('',#8146);
#2358=VERTEX_POINT('',#8150);
#2359=VERTEX_POINT('',#8152);
#2360=VERTEX_POINT('',#8156);
#2361=VERTEX_POINT('',#8158);
#2362=VERTEX_POINT('',#8162);
#2363=VERTEX_POINT('',#8164);
#2364=VERTEX_POINT('',#8168);
#2365=VERTEX_POINT('',#8170);
#2366=VERTEX_POINT('',#8174);
#2367=VERTEX_POINT('',#8176);
#2368=VERTEX_POINT('',#8180);
#2369=VERTEX_POINT('',#8182);
#2370=VERTEX_POINT('',#8186);
#2371=VERTEX_POINT('',#8188);
#2372=VERTEX_POINT('',#8192);
#2373=VERTEX_POINT('',#8194);
#2374=VERTEX_POINT('',#8198);
#2375=VERTEX_POINT('',#8199);
#2376=VERTEX_POINT('',#8201);
#2377=VERTEX_POINT('',#8203);
#2378=VERTEX_POINT('',#8207);
#2379=VERTEX_POINT('',#8209);
#2380=VERTEX_POINT('',#8213);
#2381=VERTEX_POINT('',#8215);
#2382=VERTEX_POINT('',#8219);
#2383=VERTEX_POINT('',#8221);
#2384=VERTEX_POINT('',#8225);
#2385=VERTEX_POINT('',#8227);
#2386=VERTEX_POINT('',#8231);
#2387=VERTEX_POINT('',#8233);
#2388=VERTEX_POINT('',#8237);
#2389=VERTEX_POINT('',#8239);
#2390=VERTEX_POINT('',#8243);
#2391=VERTEX_POINT('',#8245);
#2392=VERTEX_POINT('',#8249);
#2393=VERTEX_POINT('',#8251);
#2394=VERTEX_POINT('',#8255);
#2395=VERTEX_POINT('',#8257);
#2396=VERTEX_POINT('',#8261);
#2397=VERTEX_POINT('',#8263);
#2398=VERTEX_POINT('',#8267);
#2399=VERTEX_POINT('',#8269);
#2400=VERTEX_POINT('',#8273);
#2401=VERTEX_POINT('',#8275);
#2402=VERTEX_POINT('',#8279);
#2403=VERTEX_POINT('',#8281);
#2404=VERTEX_POINT('',#8285);
#2405=VERTEX_POINT('',#8287);
#2406=VERTEX_POINT('',#8294);
#2407=VERTEX_POINT('',#8296);
#2408=VERTEX_POINT('',#8300);
#2409=VERTEX_POINT('',#8302);
#2410=VERTEX_POINT('',#8309);
#2411=VERTEX_POINT('',#8311);
#2412=VERTEX_POINT('',#8315);
#2413=VERTEX_POINT('',#8317);
#2414=VERTEX_POINT('',#8330);
#2415=VERTEX_POINT('',#8332);
#2524=EDGE_CURVE('',#2054,#2055,#1084,.F.);
#2525=EDGE_CURVE('',#2056,#2055,#1085,.T.);
#2526=EDGE_CURVE('',#2057,#2056,#1086,.T.);
#2527=EDGE_CURVE('',#2054,#2057,#1087,.T.);
#2528=EDGE_CURVE('',#2054,#2058,#1088,.T.);
#2529=EDGE_CURVE('',#2059,#2057,#1089,.T.);
#2530=EDGE_CURVE('',#2058,#2059,#1090,.T.);
#2531=EDGE_CURVE('',#2058,#2060,#1091,.T.);
#2532=EDGE_CURVE('',#2061,#2059,#1092,.T.);
#2533=EDGE_CURVE('',#2060,#2061,#1093,.T.);
#2534=EDGE_CURVE('',#2062,#2055,#169,.T.);
#2535=EDGE_CURVE('',#2062,#2063,#1094,.T.);
#2536=EDGE_CURVE('',#2056,#2063,#170,.T.);
#2537=EDGE_CURVE('',#2064,#2061,#171,.T.);
#2538=EDGE_CURVE('',#2064,#2065,#1095,.T.);
#2539=EDGE_CURVE('',#2060,#2065,#172,.T.);
#2540=EDGE_CURVE('',#2066,#2067,#1096,.F.);
#2541=EDGE_CURVE('',#2068,#2067,#1097,.T.);
#2542=EDGE_CURVE('',#2069,#2068,#1098,.T.);
#2543=EDGE_CURVE('',#2066,#2069,#1099,.T.);
#2544=EDGE_CURVE('',#2066,#2070,#1100,.T.);
#2545=EDGE_CURVE('',#2071,#2069,#1101,.T.);
#2546=EDGE_CURVE('',#2070,#2071,#1102,.T.);
#2547=EDGE_CURVE('',#2070,#2072,#1103,.T.);
#2548=EDGE_CURVE('',#2073,#2071,#1104,.T.);
#2549=EDGE_CURVE('',#2072,#2073,#1105,.T.);
#2550=EDGE_CURVE('',#2074,#2067,#173,.T.);
#2551=EDGE_CURVE('',#2074,#2075,#1106,.T.);
#2552=EDGE_CURVE('',#2068,#2075,#174,.T.);
#2553=EDGE_CURVE('',#2076,#2073,#175,.T.);
#2554=EDGE_CURVE('',#2076,#2077,#1107,.T.);
#2555=EDGE_CURVE('',#2072,#2077,#176,.T.);
#2556=EDGE_CURVE('',#2078,#2065,#1108,.F.);
#2557=EDGE_CURVE('',#2079,#2064,#1109,.T.);
#2558=EDGE_CURVE('',#2078,#2079,#1110,.T.);
#2559=EDGE_CURVE('',#2078,#2080,#1111,.T.);
#2560=EDGE_CURVE('',#2081,#2079,#1112,.T.);
#2561=EDGE_CURVE('',#2080,#2081,#1113,.T.);
#2562=EDGE_CURVE('',#2080,#2082,#1114,.T.);
#2563=EDGE_CURVE('',#2083,#2081,#1115,.T.);
#2564=EDGE_CURVE('',#2082,#2083,#1116,.T.);
#2565=EDGE_CURVE('',#2084,#2083,#177,.T.);
#2566=EDGE_CURVE('',#2084,#2085,#1117,.T.);
#2567=EDGE_CURVE('',#2082,#2085,#178,.T.);
#2568=EDGE_CURVE('',#2086,#2087,#1118,.F.);
#2569=EDGE_CURVE('',#2088,#2087,#1119,.T.);
#2570=EDGE_CURVE('',#2089,#2088,#1120,.T.);
#2571=EDGE_CURVE('',#2086,#2089,#1121,.T.);
#2572=EDGE_CURVE('',#2086,#2090,#1122,.T.);
#2573=EDGE_CURVE('',#2091,#2089,#1123,.T.);
#2574=EDGE_CURVE('',#2090,#2091,#1124,.T.);
#2575=EDGE_CURVE('',#2090,#2092,#1125,.T.);
#2576=EDGE_CURVE('',#2093,#2091,#1126,.T.);
#2577=EDGE_CURVE('',#2092,#2093,#1127,.T.);
#2578=EDGE_CURVE('',#2094,#2087,#179,.T.);
#2579=EDGE_CURVE('',#2094,#2095,#1128,.T.);
#2580=EDGE_CURVE('',#2088,#2095,#180,.T.);
#2581=EDGE_CURVE('',#2096,#2093,#181,.T.);
#2582=EDGE_CURVE('',#2096,#2097,#1129,.T.);
#2583=EDGE_CURVE('',#2092,#2097,#182,.T.);
#2584=EDGE_CURVE('',#2098,#2085,#1130,.F.);
#2585=EDGE_CURVE('',#2099,#2084,#1131,.T.);
#2586=EDGE_CURVE('',#2098,#2099,#1132,.T.);
#2587=EDGE_CURVE('',#2098,#2100,#1133,.T.);
#2588=EDGE_CURVE('',#2101,#2099,#1134,.T.);
#2589=EDGE_CURVE('',#2100,#2101,#1135,.T.);
#2590=EDGE_CURVE('',#2100,#2074,#1136,.T.);
#2591=EDGE_CURVE('',#2075,#2101,#1137,.T.);
#2592=EDGE_CURVE('',#2102,#2077,#1138,.F.);
#2593=EDGE_CURVE('',#2103,#2076,#1139,.T.);
#2594=EDGE_CURVE('',#2102,#2103,#1140,.T.);
#2595=EDGE_CURVE('',#2102,#2104,#1141,.T.);
#2596=EDGE_CURVE('',#2105,#2103,#1142,.T.);
#2597=EDGE_CURVE('',#2104,#2105,#1143,.T.);
#2598=EDGE_CURVE('',#2104,#2106,#1144,.T.);
#2599=EDGE_CURVE('',#2107,#2105,#1145,.T.);
#2600=EDGE_CURVE('',#2106,#2107,#1146,.T.);
#2601=EDGE_CURVE('',#2108,#2107,#183,.T.);
#2602=EDGE_CURVE('',#2108,#2109,#1147,.T.);
#2603=EDGE_CURVE('',#2106,#2109,#184,.T.);
#2604=EDGE_CURVE('',#2110,#2111,#1148,.F.);
#2605=EDGE_CURVE('',#2112,#2111,#1149,.T.);
#2606=EDGE_CURVE('',#2113,#2112,#1150,.T.);
#2607=EDGE_CURVE('',#2110,#2113,#1151,.T.);
#2608=EDGE_CURVE('',#2110,#2114,#1152,.T.);
#2609=EDGE_CURVE('',#2115,#2113,#1153,.T.);
#2610=EDGE_CURVE('',#2114,#2115,#1154,.T.);
#2611=EDGE_CURVE('',#2114,#2062,#1155,.T.);
#2612=EDGE_CURVE('',#2063,#2115,#1156,.T.);
#2613=EDGE_CURVE('',#2116,#2111,#185,.T.);
#2614=EDGE_CURVE('',#2116,#2117,#1157,.T.);
#2615=EDGE_CURVE('',#2112,#2117,#186,.T.);
#2616=EDGE_CURVE('',#2118,#2109,#1158,.F.);
#2617=EDGE_CURVE('',#2119,#2108,#1159,.T.);
#2618=EDGE_CURVE('',#2118,#2119,#1160,.T.);
#2619=EDGE_CURVE('',#2118,#2120,#1161,.T.);
#2620=EDGE_CURVE('',#2121,#2119,#1162,.T.);
#2621=EDGE_CURVE('',#2120,#2121,#1163,.T.);
#2622=EDGE_CURVE('',#2120,#2094,#1164,.T.);
#2623=EDGE_CURVE('',#2095,#2121,#1165,.T.);
#2624=EDGE_CURVE('',#2122,#2123,#1166,.T.);
#2625=EDGE_CURVE('',#2124,#2122,#1167,.T.);
#2626=EDGE_CURVE('',#2125,#2124,#1168,.T.);
#2627=EDGE_CURVE('',#2123,#2125,#1169,.T.);
#2628=EDGE_CURVE('',#2126,#2127,#1170,.T.);
#2629=EDGE_CURVE('',#2128,#2126,#1171,.T.);
#2630=EDGE_CURVE('',#2129,#2128,#1172,.T.);
#2631=EDGE_CURVE('',#2127,#2129,#1173,.T.);
#2632=EDGE_CURVE('',#2130,#2122,#187,.T.);
#2633=EDGE_CURVE('',#2130,#2131,#1174,.T.);
#2634=EDGE_CURVE('',#2124,#2131,#188,.T.);
#2635=EDGE_CURVE('',#2132,#2129,#189,.T.);
#2636=EDGE_CURVE('',#2132,#2133,#1175,.T.);
#2637=EDGE_CURVE('',#2127,#2133,#190,.T.);
#2638=EDGE_CURVE('',#2134,#2125,#191,.T.);
#2639=EDGE_CURVE('',#2134,#2135,#1176,.T.);
#2640=EDGE_CURVE('',#2123,#2135,#192,.T.);
#2641=EDGE_CURVE('',#2136,#2126,#193,.T.);
#2642=EDGE_CURVE('',#2136,#2137,#1177,.T.);
#2643=EDGE_CURVE('',#2128,#2137,#194,.T.);
#2644=EDGE_CURVE('',#2133,#2136,#1178,.T.);
#2645=EDGE_CURVE('',#2137,#2132,#1179,.T.);
#2646=EDGE_CURVE('',#2138,#2139,#1180,.T.);
#2647=EDGE_CURVE('',#2140,#2138,#1181,.T.);
#2648=EDGE_CURVE('',#2141,#2140,#1182,.T.);
#2649=EDGE_CURVE('',#2139,#2141,#1183,.T.);
#2650=EDGE_CURVE('',#2142,#2141,#195,.T.);
#2651=EDGE_CURVE('',#2142,#2143,#1184,.T.);
#2652=EDGE_CURVE('',#2139,#2143,#196,.T.);
#2653=EDGE_CURVE('',#2144,#2138,#197,.T.);
#2654=EDGE_CURVE('',#2144,#2145,#1185,.T.);
#2655=EDGE_CURVE('',#2140,#2145,#198,.T.);
#2656=EDGE_CURVE('',#2146,#2147,#1186,.T.);
#2657=EDGE_CURVE('',#2148,#2146,#1187,.T.);
#2658=EDGE_CURVE('',#2149,#2148,#1188,.T.);
#2659=EDGE_CURVE('',#2147,#2149,#1189,.T.);
#2660=EDGE_CURVE('',#2135,#2130,#1190,.T.);
#2661=EDGE_CURVE('',#2131,#2134,#1191,.T.);
#2662=EDGE_CURVE('',#2150,#2146,#199,.T.);
#2663=EDGE_CURVE('',#2150,#2151,#1192,.T.);
#2664=EDGE_CURVE('',#2148,#2151,#200,.T.);
#2665=EDGE_CURVE('',#2152,#2149,#201,.T.);
#2666=EDGE_CURVE('',#2152,#2153,#1193,.T.);
#2667=EDGE_CURVE('',#2147,#2153,#202,.T.);
#2668=EDGE_CURVE('',#2154,#2155,#1194,.F.);
#2669=EDGE_CURVE('',#2156,#2155,#1195,.T.);
#2670=EDGE_CURVE('',#2157,#2156,#1196,.T.);
#2671=EDGE_CURVE('',#2154,#2157,#1197,.T.);
#2672=EDGE_CURVE('',#2154,#2158,#1198,.T.);
#2673=EDGE_CURVE('',#2159,#2157,#1199,.T.);
#2674=EDGE_CURVE('',#2158,#2159,#1200,.T.);
#2675=EDGE_CURVE('',#2158,#2160,#1201,.T.);
#2676=EDGE_CURVE('',#2161,#2159,#1202,.T.);
#2677=EDGE_CURVE('',#2160,#2161,#1203,.T.);
#2678=EDGE_CURVE('',#2162,#2155,#203,.T.);
#2679=EDGE_CURVE('',#2162,#2163,#1204,.T.);
#2680=EDGE_CURVE('',#2156,#2163,#204,.T.);
#2681=EDGE_CURVE('',#2164,#2161,#205,.T.);
#2682=EDGE_CURVE('',#2164,#2165,#1205,.T.);
#2683=EDGE_CURVE('',#2160,#2165,#206,.T.);
#2684=EDGE_CURVE('',#2166,#2167,#1206,.F.);
#2685=EDGE_CURVE('',#2168,#2167,#1207,.T.);
#2686=EDGE_CURVE('',#2169,#2168,#1208,.T.);
#2687=EDGE_CURVE('',#2166,#2169,#1209,.T.);
#2688=EDGE_CURVE('',#2166,#2170,#1210,.T.);
#2689=EDGE_CURVE('',#2171,#2169,#1211,.T.);
#2690=EDGE_CURVE('',#2170,#2171,#1212,.T.);
#2691=EDGE_CURVE('',#2170,#2172,#1213,.T.);
#2692=EDGE_CURVE('',#2173,#2171,#1214,.T.);
#2693=EDGE_CURVE('',#2172,#2173,#1215,.T.);
#2694=EDGE_CURVE('',#2174,#2167,#207,.T.);
#2695=EDGE_CURVE('',#2174,#2175,#1216,.T.);
#2696=EDGE_CURVE('',#2168,#2175,#208,.T.);
#2697=EDGE_CURVE('',#2176,#2173,#209,.T.);
#2698=EDGE_CURVE('',#2176,#2177,#1217,.T.);
#2699=EDGE_CURVE('',#2172,#2177,#210,.T.);
#2700=EDGE_CURVE('',#2178,#2177,#1218,.F.);
#2701=EDGE_CURVE('',#2179,#2176,#1219,.T.);
#2702=EDGE_CURVE('',#2178,#2179,#1220,.T.);
#2703=EDGE_CURVE('',#2178,#2180,#1221,.T.);
#2704=EDGE_CURVE('',#2181,#2179,#1222,.T.);
#2705=EDGE_CURVE('',#2180,#2181,#1223,.T.);
#2706=EDGE_CURVE('',#2180,#2182,#1224,.T.);
#2707=EDGE_CURVE('',#2183,#2181,#1225,.T.);
#2708=EDGE_CURVE('',#2182,#2183,#1226,.T.);
#2709=EDGE_CURVE('',#2184,#2183,#211,.T.);
#2710=EDGE_CURVE('',#2184,#2185,#1227,.T.);
#2711=EDGE_CURVE('',#2182,#2185,#212,.T.);
#2712=EDGE_CURVE('',#2186,#2185,#1228,.F.);
#2713=EDGE_CURVE('',#2187,#2184,#1229,.T.);
#2714=EDGE_CURVE('',#2186,#2187,#1230,.T.);
#2715=EDGE_CURVE('',#2186,#2188,#1231,.T.);
#2716=EDGE_CURVE('',#2189,#2187,#1232,.T.);
#2717=EDGE_CURVE('',#2188,#2189,#1233,.T.);
#2718=EDGE_CURVE('',#2188,#2162,#1234,.T.);
#2719=EDGE_CURVE('',#2163,#2189,#1235,.T.);
#2720=EDGE_CURVE('',#2190,#2165,#1236,.F.);
#2721=EDGE_CURVE('',#2191,#2164,#1237,.T.);
#2722=EDGE_CURVE('',#2190,#2191,#1238,.T.);
#2723=EDGE_CURVE('',#2190,#2192,#1239,.T.);
#2724=EDGE_CURVE('',#2193,#2191,#1240,.T.);
#2725=EDGE_CURVE('',#2192,#2193,#1241,.T.);
#2726=EDGE_CURVE('',#2192,#2194,#1242,.T.);
#2727=EDGE_CURVE('',#2195,#2193,#1243,.T.);
#2728=EDGE_CURVE('',#2194,#2195,#1244,.T.);
#2729=EDGE_CURVE('',#2196,#2195,#213,.T.);
#2730=EDGE_CURVE('',#2196,#2197,#1245,.T.);
#2731=EDGE_CURVE('',#2194,#2197,#214,.T.);
#2732=EDGE_CURVE('',#2198,#2197,#1246,.F.);
#2733=EDGE_CURVE('',#2199,#2196,#1247,.T.);
#2734=EDGE_CURVE('',#2198,#2199,#1248,.T.);
#2735=EDGE_CURVE('',#2198,#2200,#1249,.T.);
#2736=EDGE_CURVE('',#2201,#2199,#1250,.T.);
#2737=EDGE_CURVE('',#2200,#2201,#1251,.T.);
#2738=EDGE_CURVE('',#2200,#2116,#1252,.T.);
#2739=EDGE_CURVE('',#2117,#2201,#1253,.T.);
#2740=EDGE_CURVE('',#2202,#2203,#1254,.T.);
#2741=EDGE_CURVE('',#2204,#2202,#1255,.T.);
#2742=EDGE_CURVE('',#2205,#2204,#1256,.T.);
#2743=EDGE_CURVE('',#2203,#2205,#1257,.T.);
#2744=EDGE_CURVE('',#2206,#2207,#1258,.T.);
#2745=EDGE_CURVE('',#2208,#2206,#1259,.T.);
#2746=EDGE_CURVE('',#2209,#2208,#1260,.T.);
#2747=EDGE_CURVE('',#2207,#2209,#1261,.T.);
#2748=EDGE_CURVE('',#2210,#2202,#215,.T.);
#2749=EDGE_CURVE('',#2210,#2211,#1262,.T.);
#2750=EDGE_CURVE('',#2204,#2211,#216,.T.);
#2751=EDGE_CURVE('',#2212,#2209,#217,.T.);
#2752=EDGE_CURVE('',#2212,#2213,#1263,.T.);
#2753=EDGE_CURVE('',#2207,#2213,#218,.T.);
#2754=EDGE_CURVE('',#2214,#2205,#219,.T.);
#2755=EDGE_CURVE('',#2214,#2215,#1264,.T.);
#2756=EDGE_CURVE('',#2203,#2215,#220,.T.);
#2757=EDGE_CURVE('',#2216,#2206,#221,.T.);
#2758=EDGE_CURVE('',#2216,#2217,#1265,.T.);
#2759=EDGE_CURVE('',#2208,#2217,#222,.T.);
#2760=EDGE_CURVE('',#2213,#2216,#1266,.T.);
#2761=EDGE_CURVE('',#2217,#2212,#1267,.T.);
#2762=EDGE_CURVE('',#2218,#2219,#1268,.T.);
#2763=EDGE_CURVE('',#2220,#2218,#1269,.T.);
#2764=EDGE_CURVE('',#2221,#2220,#1270,.T.);
#2765=EDGE_CURVE('',#2219,#2221,#1271,.T.);
#2766=EDGE_CURVE('',#2222,#2221,#223,.T.);
#2767=EDGE_CURVE('',#2222,#2223,#1272,.T.);
#2768=EDGE_CURVE('',#2219,#2223,#224,.T.);
#2769=EDGE_CURVE('',#2224,#2218,#225,.T.);
#2770=EDGE_CURVE('',#2224,#2225,#1273,.T.);
#2771=EDGE_CURVE('',#2220,#2225,#226,.T.);
#2772=EDGE_CURVE('',#2226,#2227,#1274,.T.);
#2773=EDGE_CURVE('',#2228,#2226,#1275,.T.);
#2774=EDGE_CURVE('',#2229,#2228,#1276,.T.);
#2775=EDGE_CURVE('',#2227,#2229,#1277,.T.);
#2776=EDGE_CURVE('',#2230,#2231,#1278,.T.);
#2777=EDGE_CURVE('',#2232,#2230,#1279,.T.);
#2778=EDGE_CURVE('',#2233,#2232,#1280,.T.);
#2779=EDGE_CURVE('',#2231,#2233,#1281,.T.);
#2780=EDGE_CURVE('',#2234,#2226,#227,.T.);
#2781=EDGE_CURVE('',#2234,#2235,#1282,.T.);
#2782=EDGE_CURVE('',#2228,#2235,#228,.T.);
#2783=EDGE_CURVE('',#2236,#2233,#229,.T.);
#2784=EDGE_CURVE('',#2236,#2237,#1283,.T.);
#2785=EDGE_CURVE('',#2231,#2237,#230,.T.);
#2786=EDGE_CURVE('',#2238,#2229,#231,.T.);
#2787=EDGE_CURVE('',#2238,#2239,#1284,.T.);
#2788=EDGE_CURVE('',#2227,#2239,#232,.T.);
#2789=EDGE_CURVE('',#2240,#2230,#233,.T.);
#2790=EDGE_CURVE('',#2240,#2241,#1285,.T.);
#2791=EDGE_CURVE('',#2232,#2241,#234,.T.);
#2792=EDGE_CURVE('',#2242,#2243,#1286,.T.);
#2793=EDGE_CURVE('',#2244,#2242,#1287,.T.);
#2794=EDGE_CURVE('',#2245,#2244,#1288,.T.);
#2795=EDGE_CURVE('',#2243,#2245,#1289,.T.);
#2796=EDGE_CURVE('',#2246,#2247,#1290,.T.);
#2797=EDGE_CURVE('',#2248,#2246,#1291,.T.);
#2798=EDGE_CURVE('',#2249,#2248,#1292,.T.);
#2799=EDGE_CURVE('',#2247,#2249,#1293,.T.);
#2800=EDGE_CURVE('',#2250,#2242,#235,.T.);
#2801=EDGE_CURVE('',#2250,#2251,#1294,.T.);
#2802=EDGE_CURVE('',#2244,#2251,#236,.T.);
#2803=EDGE_CURVE('',#2252,#2249,#237,.T.);
#2804=EDGE_CURVE('',#2252,#2253,#1295,.T.);
#2805=EDGE_CURVE('',#2247,#2253,#238,.T.);
#2806=EDGE_CURVE('',#2254,#2245,#239,.T.);
#2807=EDGE_CURVE('',#2254,#2255,#1296,.T.);
#2808=EDGE_CURVE('',#2243,#2255,#240,.T.);
#2809=EDGE_CURVE('',#2256,#2246,#241,.T.);
#2810=EDGE_CURVE('',#2256,#2257,#1297,.T.);
#2811=EDGE_CURVE('',#2248,#2257,#242,.T.);
#2812=EDGE_CURVE('',#2223,#2224,#1298,.T.);
#2813=EDGE_CURVE('',#2225,#2222,#1299,.T.);
#2814=EDGE_CURVE('',#2258,#2259,#1300,.T.);
#2815=EDGE_CURVE('',#2260,#2258,#1301,.T.);
#2816=EDGE_CURVE('',#2261,#2260,#1302,.T.);
#2817=EDGE_CURVE('',#2259,#2261,#1303,.T.);
#2818=EDGE_CURVE('',#2262,#2261,#243,.T.);
#2819=EDGE_CURVE('',#2262,#2263,#1304,.T.);
#2820=EDGE_CURVE('',#2259,#2263,#244,.T.);
#2821=EDGE_CURVE('',#2264,#2258,#245,.T.);
#2822=EDGE_CURVE('',#2264,#2265,#1305,.T.);
#2823=EDGE_CURVE('',#2260,#2265,#246,.T.);
#2824=EDGE_CURVE('',#2253,#2256,#1306,.T.);
#2825=EDGE_CURVE('',#2257,#2252,#1307,.T.);
#2826=EDGE_CURVE('',#2239,#2234,#1308,.T.);
#2827=EDGE_CURVE('',#2235,#2238,#1309,.T.);
#2828=EDGE_CURVE('',#2263,#2264,#1310,.T.);
#2829=EDGE_CURVE('',#2265,#2262,#1311,.T.);
#2830=EDGE_CURVE('',#2266,#2267,#1312,.T.);
#2831=EDGE_CURVE('',#2268,#2266,#1313,.T.);
#2832=EDGE_CURVE('',#2269,#2268,#1314,.T.);
#2833=EDGE_CURVE('',#2267,#2269,#1315,.T.);
#2834=EDGE_CURVE('',#2270,#2269,#247,.T.);
#2835=EDGE_CURVE('',#2270,#2271,#1316,.T.);
#2836=EDGE_CURVE('',#2267,#2271,#248,.T.);
#2837=EDGE_CURVE('',#2272,#2266,#249,.T.);
#2838=EDGE_CURVE('',#2272,#2273,#1317,.T.);
#2839=EDGE_CURVE('',#2268,#2273,#250,.T.);
#2840=EDGE_CURVE('',#2237,#2240,#1318,.T.);
#2841=EDGE_CURVE('',#2241,#2236,#1319,.T.);
#2842=EDGE_CURVE('',#2215,#2210,#1320,.T.);
#2843=EDGE_CURVE('',#2211,#2214,#1321,.T.);
#2844=EDGE_CURVE('',#2274,#2275,#1322,.F.);
#2845=EDGE_CURVE('',#2276,#2275,#1323,.T.);
#2846=EDGE_CURVE('',#2277,#2276,#1324,.T.);
#2847=EDGE_CURVE('',#2274,#2277,#1325,.T.);
#2848=EDGE_CURVE('',#2274,#2278,#1326,.T.);
#2849=EDGE_CURVE('',#2279,#2277,#1327,.T.);
#2850=EDGE_CURVE('',#2278,#2279,#1328,.T.);
#2851=EDGE_CURVE('',#2278,#2280,#1329,.T.);
#2852=EDGE_CURVE('',#2281,#2279,#1330,.T.);
#2853=EDGE_CURVE('',#2280,#2281,#1331,.T.);
#2854=EDGE_CURVE('',#2282,#2275,#251,.T.);
#2855=EDGE_CURVE('',#2282,#2283,#1332,.T.);
#2856=EDGE_CURVE('',#2276,#2283,#252,.T.);
#2857=EDGE_CURVE('',#2284,#2281,#253,.T.);
#2858=EDGE_CURVE('',#2284,#2285,#1333,.T.);
#2859=EDGE_CURVE('',#2280,#2285,#254,.T.);
#2860=EDGE_CURVE('',#2286,#2285,#1334,.F.);
#2861=EDGE_CURVE('',#2287,#2284,#1335,.T.);
#2862=EDGE_CURVE('',#2286,#2287,#1336,.T.);
#2863=EDGE_CURVE('',#2286,#2288,#1337,.T.);
#2864=EDGE_CURVE('',#2289,#2287,#1338,.T.);
#2865=EDGE_CURVE('',#2288,#2289,#1339,.T.);
#2866=EDGE_CURVE('',#2288,#2290,#1340,.T.);
#2867=EDGE_CURVE('',#2291,#2289,#1341,.T.);
#2868=EDGE_CURVE('',#2290,#2291,#1342,.T.);
#2869=EDGE_CURVE('',#2292,#2291,#255,.T.);
#2870=EDGE_CURVE('',#2292,#2293,#1343,.T.);
#2871=EDGE_CURVE('',#2290,#2293,#256,.T.);
#2872=EDGE_CURVE('',#2294,#2295,#1344,.F.);
#2873=EDGE_CURVE('',#2296,#2295,#1345,.T.);
#2874=EDGE_CURVE('',#2297,#2296,#1346,.T.);
#2875=EDGE_CURVE('',#2294,#2297,#1347,.T.);
#2876=EDGE_CURVE('',#2294,#2298,#1348,.T.);
#2877=EDGE_CURVE('',#2299,#2297,#1349,.T.);
#2878=EDGE_CURVE('',#2298,#2299,#1350,.T.);
#2879=EDGE_CURVE('',#2298,#2300,#1351,.T.);
#2880=EDGE_CURVE('',#2301,#2299,#1352,.T.);
#2881=EDGE_CURVE('',#2300,#2301,#1353,.T.);
#2882=EDGE_CURVE('',#2302,#2295,#257,.T.);
#2883=EDGE_CURVE('',#2302,#2303,#1354,.T.);
#2884=EDGE_CURVE('',#2296,#2303,#258,.T.);
#2885=EDGE_CURVE('',#2304,#2301,#259,.T.);
#2886=EDGE_CURVE('',#2304,#2305,#1355,.T.);
#2887=EDGE_CURVE('',#2300,#2305,#260,.T.);
#2888=EDGE_CURVE('',#2306,#2307,#1356,.F.);
#2889=EDGE_CURVE('',#2308,#2307,#1357,.T.);
#2890=EDGE_CURVE('',#2309,#2308,#1358,.T.);
#2891=EDGE_CURVE('',#2306,#2309,#1359,.T.);
#2892=EDGE_CURVE('',#2306,#2310,#1360,.T.);
#2893=EDGE_CURVE('',#2311,#2309,#1361,.T.);
#2894=EDGE_CURVE('',#2310,#2311,#1362,.T.);
#2895=EDGE_CURVE('',#2310,#2312,#1363,.T.);
#2896=EDGE_CURVE('',#2313,#2311,#1364,.T.);
#2897=EDGE_CURVE('',#2312,#2313,#1365,.T.);
#2898=EDGE_CURVE('',#2314,#2307,#261,.T.);
#2899=EDGE_CURVE('',#2314,#2315,#1366,.T.);
#2900=EDGE_CURVE('',#2308,#2315,#262,.T.);
#2901=EDGE_CURVE('',#2316,#2313,#263,.T.);
#2902=EDGE_CURVE('',#2316,#2317,#1367,.T.);
#2903=EDGE_CURVE('',#2312,#2317,#264,.T.);
#2904=EDGE_CURVE('',#2318,#2305,#1368,.F.);
#2905=EDGE_CURVE('',#2319,#2304,#1369,.T.);
#2906=EDGE_CURVE('',#2318,#2319,#1370,.T.);
#2907=EDGE_CURVE('',#2318,#2320,#1371,.T.);
#2908=EDGE_CURVE('',#2321,#2319,#1372,.T.);
#2909=EDGE_CURVE('',#2320,#2321,#1373,.T.);
#2910=EDGE_CURVE('',#2320,#2314,#1374,.T.);
#2911=EDGE_CURVE('',#2315,#2321,#1375,.T.);
#2912=EDGE_CURVE('',#2322,#2097,#1376,.F.);
#2913=EDGE_CURVE('',#2323,#2096,#1377,.T.);
#2914=EDGE_CURVE('',#2322,#2323,#1378,.T.);
#2915=EDGE_CURVE('',#2322,#2324,#1379,.T.);
#2916=EDGE_CURVE('',#2325,#2323,#1380,.T.);
#2917=EDGE_CURVE('',#2324,#2325,#1381,.T.);
#2918=EDGE_CURVE('',#2324,#2282,#1382,.T.);
#2919=EDGE_CURVE('',#2283,#2325,#1383,.T.);
#2920=EDGE_CURVE('',#2326,#2293,#1384,.F.);
#2921=EDGE_CURVE('',#2327,#2292,#1385,.T.);
#2922=EDGE_CURVE('',#2326,#2327,#1386,.T.);
#2923=EDGE_CURVE('',#2326,#2328,#1387,.T.);
#2924=EDGE_CURVE('',#2329,#2327,#1388,.T.);
#2925=EDGE_CURVE('',#2328,#2329,#1389,.T.);
#2926=EDGE_CURVE('',#2328,#2302,#1390,.T.);
#2927=EDGE_CURVE('',#2303,#2329,#1391,.T.);
#2928=EDGE_CURVE('',#2330,#2317,#1392,.F.);
#2929=EDGE_CURVE('',#2331,#2316,#1393,.T.);
#2930=EDGE_CURVE('',#2330,#2331,#1394,.T.);
#2931=EDGE_CURVE('',#2330,#2332,#1395,.T.);
#2932=EDGE_CURVE('',#2333,#2331,#1396,.T.);
#2933=EDGE_CURVE('',#2332,#2333,#1397,.T.);
#2934=EDGE_CURVE('',#2332,#2334,#1398,.T.);
#2935=EDGE_CURVE('',#2335,#2333,#1399,.T.);
#2936=EDGE_CURVE('',#2334,#2335,#1400,.T.);
#2937=EDGE_CURVE('',#2336,#2335,#265,.T.);
#2938=EDGE_CURVE('',#2336,#2337,#1401,.T.);
#2939=EDGE_CURVE('',#2334,#2337,#266,.T.);
#2940=EDGE_CURVE('',#2271,#2272,#1402,.T.);
#2941=EDGE_CURVE('',#2273,#2270,#1403,.T.);
#2942=EDGE_CURVE('',#2338,#2339,#1404,.T.);
#2943=EDGE_CURVE('',#2340,#2338,#1405,.T.);
#2944=EDGE_CURVE('',#2341,#2340,#1406,.T.);
#2945=EDGE_CURVE('',#2339,#2341,#1407,.T.);
#2946=EDGE_CURVE('',#2342,#2341,#267,.T.);
#2947=EDGE_CURVE('',#2342,#2343,#1408,.T.);
#2948=EDGE_CURVE('',#2339,#2343,#268,.T.);
#2949=EDGE_CURVE('',#2344,#2338,#269,.T.);
#2950=EDGE_CURVE('',#2344,#2345,#1409,.T.);
#2951=EDGE_CURVE('',#2340,#2345,#270,.T.);
#2952=EDGE_CURVE('',#2346,#2347,#1410,.T.);
#2953=EDGE_CURVE('',#2348,#2346,#1411,.T.);
#2954=EDGE_CURVE('',#2349,#2348,#1412,.T.);
#2955=EDGE_CURVE('',#2347,#2349,#1413,.T.);
#2956=EDGE_CURVE('',#2153,#2150,#1414,.T.);
#2957=EDGE_CURVE('',#2151,#2152,#1415,.T.);
#2958=EDGE_CURVE('',#2350,#2346,#271,.T.);
#2959=EDGE_CURVE('',#2350,#2351,#1416,.T.);
#2960=EDGE_CURVE('',#2348,#2351,#272,.T.);
#2961=EDGE_CURVE('',#2352,#2349,#273,.T.);
#2962=EDGE_CURVE('',#2352,#2353,#1417,.T.);
#2963=EDGE_CURVE('',#2347,#2353,#274,.T.);
#2964=EDGE_CURVE('',#2343,#2344,#1418,.T.);
#2965=EDGE_CURVE('',#2345,#2342,#1419,.T.);
#2966=EDGE_CURVE('',#2353,#2350,#1420,.T.);
#2967=EDGE_CURVE('',#2351,#2352,#1421,.T.);
#2968=EDGE_CURVE('',#2354,#2355,#1422,.F.);
#2969=EDGE_CURVE('',#2356,#2355,#1423,.T.);
#2970=EDGE_CURVE('',#2357,#2356,#1424,.T.);
#2971=EDGE_CURVE('',#2354,#2357,#1425,.T.);
#2972=EDGE_CURVE('',#2354,#2358,#1426,.T.);
#2973=EDGE_CURVE('',#2359,#2357,#1427,.T.);
#2974=EDGE_CURVE('',#2358,#2359,#1428,.T.);
#2975=EDGE_CURVE('',#2358,#2360,#1429,.T.);
#2976=EDGE_CURVE('',#2361,#2359,#1430,.T.);
#2977=EDGE_CURVE('',#2360,#2361,#1431,.T.);
#2978=EDGE_CURVE('',#2362,#2355,#275,.T.);
#2979=EDGE_CURVE('',#2362,#2363,#1432,.T.);
#2980=EDGE_CURVE('',#2356,#2363,#276,.T.);
#2981=EDGE_CURVE('',#2364,#2361,#277,.T.);
#2982=EDGE_CURVE('',#2364,#2365,#1433,.T.);
#2983=EDGE_CURVE('',#2360,#2365,#278,.T.);
#2984=EDGE_CURVE('',#2366,#2365,#1434,.F.);
#2985=EDGE_CURVE('',#2367,#2364,#1435,.T.);
#2986=EDGE_CURVE('',#2366,#2367,#1436,.T.);
#2987=EDGE_CURVE('',#2366,#2368,#1437,.T.);
#2988=EDGE_CURVE('',#2369,#2367,#1438,.T.);
#2989=EDGE_CURVE('',#2368,#2369,#1439,.T.);
#2990=EDGE_CURVE('',#2368,#2370,#1440,.T.);
#2991=EDGE_CURVE('',#2371,#2369,#1441,.T.);
#2992=EDGE_CURVE('',#2370,#2371,#1442,.T.);
#2993=EDGE_CURVE('',#2372,#2371,#279,.T.);
#2994=EDGE_CURVE('',#2372,#2373,#1443,.T.);
#2995=EDGE_CURVE('',#2370,#2373,#280,.T.);
#2996=EDGE_CURVE('',#2374,#2375,#1444,.F.);
#2997=EDGE_CURVE('',#2376,#2375,#1445,.T.);
#2998=EDGE_CURVE('',#2377,#2376,#1446,.T.);
#2999=EDGE_CURVE('',#2374,#2377,#1447,.T.);
#3000=EDGE_CURVE('',#2374,#2378,#1448,.T.);
#3001=EDGE_CURVE('',#2379,#2377,#1449,.T.);
#3002=EDGE_CURVE('',#2378,#2379,#1450,.T.);
#3003=EDGE_CURVE('',#2378,#2380,#1451,.T.);
#3004=EDGE_CURVE('',#2381,#2379,#1452,.T.);
#3005=EDGE_CURVE('',#2380,#2381,#1453,.T.);
#3006=EDGE_CURVE('',#2382,#2375,#281,.T.);
#3007=EDGE_CURVE('',#2382,#2383,#1454,.T.);
#3008=EDGE_CURVE('',#2376,#2383,#282,.T.);
#3009=EDGE_CURVE('',#2384,#2381,#283,.T.);
#3010=EDGE_CURVE('',#2384,#2385,#1455,.T.);
#3011=EDGE_CURVE('',#2380,#2385,#284,.T.);
#3012=EDGE_CURVE('',#2386,#2373,#1456,.F.);
#3013=EDGE_CURVE('',#2387,#2372,#1457,.T.);
#3014=EDGE_CURVE('',#2386,#2387,#1458,.T.);
#3015=EDGE_CURVE('',#2386,#2388,#1459,.T.);
#3016=EDGE_CURVE('',#2389,#2387,#1460,.T.);
#3017=EDGE_CURVE('',#2388,#2389,#1461,.T.);
#3018=EDGE_CURVE('',#2388,#2390,#1462,.T.);
#3019=EDGE_CURVE('',#2391,#2389,#1463,.T.);
#3020=EDGE_CURVE('',#2390,#2391,#1464,.T.);
#3021=EDGE_CURVE('',#2392,#2391,#285,.T.);
#3022=EDGE_CURVE('',#2392,#2393,#1465,.T.);
#3023=EDGE_CURVE('',#2390,#2393,#286,.T.);
#3024=EDGE_CURVE('',#2394,#2337,#1466,.F.);
#3025=EDGE_CURVE('',#2395,#2336,#1467,.T.);
#3026=EDGE_CURVE('',#2394,#2395,#1468,.T.);
#3027=EDGE_CURVE('',#2394,#2396,#1469,.T.);
#3028=EDGE_CURVE('',#2397,#2395,#1470,.T.);
#3029=EDGE_CURVE('',#2396,#2397,#1471,.T.);
#3030=EDGE_CURVE('',#2396,#2398,#1472,.T.);
#3031=EDGE_CURVE('',#2399,#2397,#1473,.T.);
#3032=EDGE_CURVE('',#2398,#2399,#1474,.T.);
#3033=EDGE_CURVE('',#2400,#2399,#287,.T.);
#3034=EDGE_CURVE('',#2400,#2401,#1475,.T.);
#3035=EDGE_CURVE('',#2398,#2401,#288,.T.);
#3036=EDGE_CURVE('',#2402,#2385,#1476,.F.);
#3037=EDGE_CURVE('',#2403,#2384,#1477,.T.);
#3038=EDGE_CURVE('',#2402,#2403,#1478,.T.);
#3039=EDGE_CURVE('',#2402,#2404,#1479,.T.);
#3040=EDGE_CURVE('',#2405,#2403,#1480,.T.);
#3041=EDGE_CURVE('',#2404,#2405,#1481,.T.);
#3042=EDGE_CURVE('',#2404,#2174,#1482,.T.);
#3043=EDGE_CURVE('',#2175,#2405,#1483,.T.);
#3044=EDGE_CURVE('',#2406,#2393,#1484,.F.);
#3045=EDGE_CURVE('',#2407,#2392,#1485,.T.);
#3046=EDGE_CURVE('',#2406,#2407,#1486,.T.);
#3047=EDGE_CURVE('',#2406,#2408,#1487,.T.);
#3048=EDGE_CURVE('',#2409,#2407,#1488,.T.);
#3049=EDGE_CURVE('',#2408,#2409,#1489,.T.);
#3050=EDGE_CURVE('',#2408,#2382,#1490,.T.);
#3051=EDGE_CURVE('',#2383,#2409,#1491,.T.);
#3052=EDGE_CURVE('',#2410,#2401,#1492,.F.);
#3053=EDGE_CURVE('',#2411,#2400,#1493,.T.);
#3054=EDGE_CURVE('',#2410,#2411,#1494,.T.);
#3055=EDGE_CURVE('',#2410,#2412,#1495,.T.);
#3056=EDGE_CURVE('',#2413,#2411,#1496,.T.);
#3057=EDGE_CURVE('',#2412,#2413,#1497,.T.);
#3058=EDGE_CURVE('',#2412,#2362,#1498,.T.);
#3059=EDGE_CURVE('',#2363,#2413,#1499,.T.);
#3060=EDGE_CURVE('',#2143,#2144,#1500,.T.);
#3061=EDGE_CURVE('',#2145,#2142,#1501,.T.);
#3062=EDGE_CURVE('',#2255,#2250,#1502,.T.);
#3063=EDGE_CURVE('',#2251,#2254,#1503,.T.);
#3064=EDGE_CURVE('',#2414,#2414,#289,.T.);
#3065=EDGE_CURVE('',#2414,#2415,#1504,.T.);
#3066=EDGE_CURVE('',#2415,#2415,#290,.T.);
#3240=ORIENTED_EDGE('',*,*,#2524,.T.);
#3241=ORIENTED_EDGE('',*,*,#2525,.F.);
#3242=ORIENTED_EDGE('',*,*,#2526,.F.);
#3243=ORIENTED_EDGE('',*,*,#2527,.F.);
#3244=ORIENTED_EDGE('',*,*,#2528,.F.);
#3245=ORIENTED_EDGE('',*,*,#2527,.T.);
#3246=ORIENTED_EDGE('',*,*,#2529,.F.);
#3247=ORIENTED_EDGE('',*,*,#2530,.F.);
#3248=ORIENTED_EDGE('',*,*,#2531,.F.);
#3249=ORIENTED_EDGE('',*,*,#2530,.T.);
#3250=ORIENTED_EDGE('',*,*,#2532,.F.);
#3251=ORIENTED_EDGE('',*,*,#2533,.F.);
#3252=ORIENTED_EDGE('',*,*,#2525,.T.);
#3253=ORIENTED_EDGE('',*,*,#2534,.F.);
#3254=ORIENTED_EDGE('',*,*,#2535,.T.);
#3255=ORIENTED_EDGE('',*,*,#2536,.F.);
#3256=ORIENTED_EDGE('',*,*,#2533,.T.);
#3257=ORIENTED_EDGE('',*,*,#2537,.F.);
#3258=ORIENTED_EDGE('',*,*,#2538,.T.);
#3259=ORIENTED_EDGE('',*,*,#2539,.F.);
#3260=ORIENTED_EDGE('',*,*,#2540,.T.);
#3261=ORIENTED_EDGE('',*,*,#2541,.F.);
#3262=ORIENTED_EDGE('',*,*,#2542,.F.);
#3263=ORIENTED_EDGE('',*,*,#2543,.F.);
#3264=ORIENTED_EDGE('',*,*,#2544,.F.);
#3265=ORIENTED_EDGE('',*,*,#2543,.T.);
#3266=ORIENTED_EDGE('',*,*,#2545,.F.);
#3267=ORIENTED_EDGE('',*,*,#2546,.F.);
#3268=ORIENTED_EDGE('',*,*,#2547,.F.);
#3269=ORIENTED_EDGE('',*,*,#2546,.T.);
#3270=ORIENTED_EDGE('',*,*,#2548,.F.);
#3271=ORIENTED_EDGE('',*,*,#2549,.F.);
#3272=ORIENTED_EDGE('',*,*,#2541,.T.);
#3273=ORIENTED_EDGE('',*,*,#2550,.F.);
#3274=ORIENTED_EDGE('',*,*,#2551,.T.);
#3275=ORIENTED_EDGE('',*,*,#2552,.F.);
#3276=ORIENTED_EDGE('',*,*,#2549,.T.);
#3277=ORIENTED_EDGE('',*,*,#2553,.F.);
#3278=ORIENTED_EDGE('',*,*,#2554,.T.);
#3279=ORIENTED_EDGE('',*,*,#2555,.F.);
#3280=ORIENTED_EDGE('',*,*,#2556,.T.);
#3281=ORIENTED_EDGE('',*,*,#2538,.F.);
#3282=ORIENTED_EDGE('',*,*,#2557,.F.);
#3283=ORIENTED_EDGE('',*,*,#2558,.F.);
#3284=ORIENTED_EDGE('',*,*,#2559,.F.);
#3285=ORIENTED_EDGE('',*,*,#2558,.T.);
#3286=ORIENTED_EDGE('',*,*,#2560,.F.);
#3287=ORIENTED_EDGE('',*,*,#2561,.F.);
#3288=ORIENTED_EDGE('',*,*,#2562,.F.);
#3289=ORIENTED_EDGE('',*,*,#2561,.T.);
#3290=ORIENTED_EDGE('',*,*,#2563,.F.);
#3291=ORIENTED_EDGE('',*,*,#2564,.F.);
#3292=ORIENTED_EDGE('',*,*,#2564,.T.);
#3293=ORIENTED_EDGE('',*,*,#2565,.F.);
#3294=ORIENTED_EDGE('',*,*,#2566,.T.);
#3295=ORIENTED_EDGE('',*,*,#2567,.F.);
#3296=ORIENTED_EDGE('',*,*,#2568,.T.);
#3297=ORIENTED_EDGE('',*,*,#2569,.F.);
#3298=ORIENTED_EDGE('',*,*,#2570,.F.);
#3299=ORIENTED_EDGE('',*,*,#2571,.F.);
#3300=ORIENTED_EDGE('',*,*,#2572,.F.);
#3301=ORIENTED_EDGE('',*,*,#2571,.T.);
#3302=ORIENTED_EDGE('',*,*,#2573,.F.);
#3303=ORIENTED_EDGE('',*,*,#2574,.F.);
#3304=ORIENTED_EDGE('',*,*,#2575,.F.);
#3305=ORIENTED_EDGE('',*,*,#2574,.T.);
#3306=ORIENTED_EDGE('',*,*,#2576,.F.);
#3307=ORIENTED_EDGE('',*,*,#2577,.F.);
#3308=ORIENTED_EDGE('',*,*,#2569,.T.);
#3309=ORIENTED_EDGE('',*,*,#2578,.F.);
#3310=ORIENTED_EDGE('',*,*,#2579,.T.);
#3311=ORIENTED_EDGE('',*,*,#2580,.F.);
#3312=ORIENTED_EDGE('',*,*,#2577,.T.);
#3313=ORIENTED_EDGE('',*,*,#2581,.F.);
#3314=ORIENTED_EDGE('',*,*,#2582,.T.);
#3315=ORIENTED_EDGE('',*,*,#2583,.F.);
#3316=ORIENTED_EDGE('',*,*,#2584,.T.);
#3317=ORIENTED_EDGE('',*,*,#2566,.F.);
#3318=ORIENTED_EDGE('',*,*,#2585,.F.);
#3319=ORIENTED_EDGE('',*,*,#2586,.F.);
#3320=ORIENTED_EDGE('',*,*,#2587,.F.);
#3321=ORIENTED_EDGE('',*,*,#2586,.T.);
#3322=ORIENTED_EDGE('',*,*,#2588,.F.);
#3323=ORIENTED_EDGE('',*,*,#2589,.F.);
#3324=ORIENTED_EDGE('',*,*,#2590,.F.);
#3325=ORIENTED_EDGE('',*,*,#2589,.T.);
#3326=ORIENTED_EDGE('',*,*,#2591,.F.);
#3327=ORIENTED_EDGE('',*,*,#2551,.F.);
#3328=ORIENTED_EDGE('',*,*,#2592,.T.);
#3329=ORIENTED_EDGE('',*,*,#2554,.F.);
#3330=ORIENTED_EDGE('',*,*,#2593,.F.);
#3331=ORIENTED_EDGE('',*,*,#2594,.F.);
#3332=ORIENTED_EDGE('',*,*,#2595,.F.);
#3333=ORIENTED_EDGE('',*,*,#2594,.T.);
#3334=ORIENTED_EDGE('',*,*,#2596,.F.);
#3335=ORIENTED_EDGE('',*,*,#2597,.F.);
#3336=ORIENTED_EDGE('',*,*,#2598,.F.);
#3337=ORIENTED_EDGE('',*,*,#2597,.T.);
#3338=ORIENTED_EDGE('',*,*,#2599,.F.);
#3339=ORIENTED_EDGE('',*,*,#2600,.F.);
#3340=ORIENTED_EDGE('',*,*,#2600,.T.);
#3341=ORIENTED_EDGE('',*,*,#2601,.F.);
#3342=ORIENTED_EDGE('',*,*,#2602,.T.);
#3343=ORIENTED_EDGE('',*,*,#2603,.F.);
#3344=ORIENTED_EDGE('',*,*,#2604,.T.);
#3345=ORIENTED_EDGE('',*,*,#2605,.F.);
#3346=ORIENTED_EDGE('',*,*,#2606,.F.);
#3347=ORIENTED_EDGE('',*,*,#2607,.F.);
#3348=ORIENTED_EDGE('',*,*,#2608,.F.);
#3349=ORIENTED_EDGE('',*,*,#2607,.T.);
#3350=ORIENTED_EDGE('',*,*,#2609,.F.);
#3351=ORIENTED_EDGE('',*,*,#2610,.F.);
#3352=ORIENTED_EDGE('',*,*,#2611,.F.);
#3353=ORIENTED_EDGE('',*,*,#2610,.T.);
#3354=ORIENTED_EDGE('',*,*,#2612,.F.);
#3355=ORIENTED_EDGE('',*,*,#2535,.F.);
#3356=ORIENTED_EDGE('',*,*,#2605,.T.);
#3357=ORIENTED_EDGE('',*,*,#2613,.F.);
#3358=ORIENTED_EDGE('',*,*,#2614,.T.);
#3359=ORIENTED_EDGE('',*,*,#2615,.F.);
#3360=ORIENTED_EDGE('',*,*,#2616,.T.);
#3361=ORIENTED_EDGE('',*,*,#2602,.F.);
#3362=ORIENTED_EDGE('',*,*,#2617,.F.);
#3363=ORIENTED_EDGE('',*,*,#2618,.F.);
#3364=ORIENTED_EDGE('',*,*,#2619,.F.);
#3365=ORIENTED_EDGE('',*,*,#2618,.T.);
#3366=ORIENTED_EDGE('',*,*,#2620,.F.);
#3367=ORIENTED_EDGE('',*,*,#2621,.F.);
#3368=ORIENTED_EDGE('',*,*,#2622,.F.);
#3369=ORIENTED_EDGE('',*,*,#2621,.T.);
#3370=ORIENTED_EDGE('',*,*,#2623,.F.);
#3371=ORIENTED_EDGE('',*,*,#2579,.F.);
#3372=ORIENTED_EDGE('',*,*,#2624,.F.);
#3373=ORIENTED_EDGE('',*,*,#2625,.F.);
#3374=ORIENTED_EDGE('',*,*,#2626,.F.);
#3375=ORIENTED_EDGE('',*,*,#2627,.F.);
#3376=ORIENTED_EDGE('',*,*,#2628,.F.);
#3377=ORIENTED_EDGE('',*,*,#2629,.F.);
#3378=ORIENTED_EDGE('',*,*,#2630,.F.);
#3379=ORIENTED_EDGE('',*,*,#2631,.F.);
#3380=ORIENTED_EDGE('',*,*,#2625,.T.);
#3381=ORIENTED_EDGE('',*,*,#2632,.F.);
#3382=ORIENTED_EDGE('',*,*,#2633,.T.);
#3383=ORIENTED_EDGE('',*,*,#2634,.F.);
#3384=ORIENTED_EDGE('',*,*,#2631,.T.);
#3385=ORIENTED_EDGE('',*,*,#2635,.F.);
#3386=ORIENTED_EDGE('',*,*,#2636,.T.);
#3387=ORIENTED_EDGE('',*,*,#2637,.F.);
#3388=ORIENTED_EDGE('',*,*,#2627,.T.);
#3389=ORIENTED_EDGE('',*,*,#2638,.F.);
#3390=ORIENTED_EDGE('',*,*,#2639,.T.);
#3391=ORIENTED_EDGE('',*,*,#2640,.F.);
#3392=ORIENTED_EDGE('',*,*,#2629,.T.);
#3393=ORIENTED_EDGE('',*,*,#2641,.F.);
#3394=ORIENTED_EDGE('',*,*,#2642,.T.);
#3395=ORIENTED_EDGE('',*,*,#2643,.F.);
#3396=ORIENTED_EDGE('',*,*,#2644,.F.);
#3397=ORIENTED_EDGE('',*,*,#2636,.F.);
#3398=ORIENTED_EDGE('',*,*,#2645,.F.);
#3399=ORIENTED_EDGE('',*,*,#2642,.F.);
#3400=ORIENTED_EDGE('',*,*,#2646,.F.);
#3401=ORIENTED_EDGE('',*,*,#2647,.F.);
#3402=ORIENTED_EDGE('',*,*,#2648,.F.);
#3403=ORIENTED_EDGE('',*,*,#2649,.F.);
#3404=ORIENTED_EDGE('',*,*,#2649,.T.);
#3405=ORIENTED_EDGE('',*,*,#2650,.F.);
#3406=ORIENTED_EDGE('',*,*,#2651,.T.);
#3407=ORIENTED_EDGE('',*,*,#2652,.F.);
#3408=ORIENTED_EDGE('',*,*,#2647,.T.);
#3409=ORIENTED_EDGE('',*,*,#2653,.F.);
#3410=ORIENTED_EDGE('',*,*,#2654,.T.);
#3411=ORIENTED_EDGE('',*,*,#2655,.F.);
#3412=ORIENTED_EDGE('',*,*,#2656,.F.);
#3413=ORIENTED_EDGE('',*,*,#2657,.F.);
#3414=ORIENTED_EDGE('',*,*,#2658,.F.);
#3415=ORIENTED_EDGE('',*,*,#2659,.F.);
#3416=ORIENTED_EDGE('',*,*,#2660,.F.);
#3417=ORIENTED_EDGE('',*,*,#2639,.F.);
#3418=ORIENTED_EDGE('',*,*,#2661,.F.);
#3419=ORIENTED_EDGE('',*,*,#2633,.F.);
#3420=ORIENTED_EDGE('',*,*,#2657,.T.);
#3421=ORIENTED_EDGE('',*,*,#2662,.F.);
#3422=ORIENTED_EDGE('',*,*,#2663,.T.);
#3423=ORIENTED_EDGE('',*,*,#2664,.F.);
#3424=ORIENTED_EDGE('',*,*,#2659,.T.);
#3425=ORIENTED_EDGE('',*,*,#2665,.F.);
#3426=ORIENTED_EDGE('',*,*,#2666,.T.);
#3427=ORIENTED_EDGE('',*,*,#2667,.F.);
#3428=ORIENTED_EDGE('',*,*,#2668,.T.);
#3429=ORIENTED_EDGE('',*,*,#2669,.F.);
#3430=ORIENTED_EDGE('',*,*,#2670,.F.);
#3431=ORIENTED_EDGE('',*,*,#2671,.F.);
#3432=ORIENTED_EDGE('',*,*,#2672,.F.);
#3433=ORIENTED_EDGE('',*,*,#2671,.T.);
#3434=ORIENTED_EDGE('',*,*,#2673,.F.);
#3435=ORIENTED_EDGE('',*,*,#2674,.F.);
#3436=ORIENTED_EDGE('',*,*,#2675,.F.);
#3437=ORIENTED_EDGE('',*,*,#2674,.T.);
#3438=ORIENTED_EDGE('',*,*,#2676,.F.);
#3439=ORIENTED_EDGE('',*,*,#2677,.F.);
#3440=ORIENTED_EDGE('',*,*,#2669,.T.);
#3441=ORIENTED_EDGE('',*,*,#2678,.F.);
#3442=ORIENTED_EDGE('',*,*,#2679,.T.);
#3443=ORIENTED_EDGE('',*,*,#2680,.F.);
#3444=ORIENTED_EDGE('',*,*,#2677,.T.);
#3445=ORIENTED_EDGE('',*,*,#2681,.F.);
#3446=ORIENTED_EDGE('',*,*,#2682,.T.);
#3447=ORIENTED_EDGE('',*,*,#2683,.F.);
#3448=ORIENTED_EDGE('',*,*,#2684,.T.);
#3449=ORIENTED_EDGE('',*,*,#2685,.F.);
#3450=ORIENTED_EDGE('',*,*,#2686,.F.);
#3451=ORIENTED_EDGE('',*,*,#2687,.F.);
#3452=ORIENTED_EDGE('',*,*,#2688,.F.);
#3453=ORIENTED_EDGE('',*,*,#2687,.T.);
#3454=ORIENTED_EDGE('',*,*,#2689,.F.);
#3455=ORIENTED_EDGE('',*,*,#2690,.F.);
#3456=ORIENTED_EDGE('',*,*,#2691,.F.);
#3457=ORIENTED_EDGE('',*,*,#2690,.T.);
#3458=ORIENTED_EDGE('',*,*,#2692,.F.);
#3459=ORIENTED_EDGE('',*,*,#2693,.F.);
#3460=ORIENTED_EDGE('',*,*,#2685,.T.);
#3461=ORIENTED_EDGE('',*,*,#2694,.F.);
#3462=ORIENTED_EDGE('',*,*,#2695,.T.);
#3463=ORIENTED_EDGE('',*,*,#2696,.F.);
#3464=ORIENTED_EDGE('',*,*,#2693,.T.);
#3465=ORIENTED_EDGE('',*,*,#2697,.F.);
#3466=ORIENTED_EDGE('',*,*,#2698,.T.);
#3467=ORIENTED_EDGE('',*,*,#2699,.F.);
#3468=ORIENTED_EDGE('',*,*,#2700,.T.);
#3469=ORIENTED_EDGE('',*,*,#2698,.F.);
#3470=ORIENTED_EDGE('',*,*,#2701,.F.);
#3471=ORIENTED_EDGE('',*,*,#2702,.F.);
#3472=ORIENTED_EDGE('',*,*,#2703,.F.);
#3473=ORIENTED_EDGE('',*,*,#2702,.T.);
#3474=ORIENTED_EDGE('',*,*,#2704,.F.);
#3475=ORIENTED_EDGE('',*,*,#2705,.F.);
#3476=ORIENTED_EDGE('',*,*,#2706,.F.);
#3477=ORIENTED_EDGE('',*,*,#2705,.T.);
#3478=ORIENTED_EDGE('',*,*,#2707,.F.);
#3479=ORIENTED_EDGE('',*,*,#2708,.F.);
#3480=ORIENTED_EDGE('',*,*,#2708,.T.);
#3481=ORIENTED_EDGE('',*,*,#2709,.F.);
#3482=ORIENTED_EDGE('',*,*,#2710,.T.);
#3483=ORIENTED_EDGE('',*,*,#2711,.F.);
#3484=ORIENTED_EDGE('',*,*,#2712,.T.);
#3485=ORIENTED_EDGE('',*,*,#2710,.F.);
#3486=ORIENTED_EDGE('',*,*,#2713,.F.);
#3487=ORIENTED_EDGE('',*,*,#2714,.F.);
#3488=ORIENTED_EDGE('',*,*,#2715,.F.);
#3489=ORIENTED_EDGE('',*,*,#2714,.T.);
#3490=ORIENTED_EDGE('',*,*,#2716,.F.);
#3491=ORIENTED_EDGE('',*,*,#2717,.F.);
#3492=ORIENTED_EDGE('',*,*,#2718,.F.);
#3493=ORIENTED_EDGE('',*,*,#2717,.T.);
#3494=ORIENTED_EDGE('',*,*,#2719,.F.);
#3495=ORIENTED_EDGE('',*,*,#2679,.F.);
#3496=ORIENTED_EDGE('',*,*,#2720,.T.);
#3497=ORIENTED_EDGE('',*,*,#2682,.F.);
#3498=ORIENTED_EDGE('',*,*,#2721,.F.);
#3499=ORIENTED_EDGE('',*,*,#2722,.F.);
#3500=ORIENTED_EDGE('',*,*,#2723,.F.);
#3501=ORIENTED_EDGE('',*,*,#2722,.T.);
#3502=ORIENTED_EDGE('',*,*,#2724,.F.);
#3503=ORIENTED_EDGE('',*,*,#2725,.F.);
#3504=ORIENTED_EDGE('',*,*,#2726,.F.);
#3505=ORIENTED_EDGE('',*,*,#2725,.T.);
#3506=ORIENTED_EDGE('',*,*,#2727,.F.);
#3507=ORIENTED_EDGE('',*,*,#2728,.F.);
#3508=ORIENTED_EDGE('',*,*,#2728,.T.);
#3509=ORIENTED_EDGE('',*,*,#2729,.F.);
#3510=ORIENTED_EDGE('',*,*,#2730,.T.);
#3511=ORIENTED_EDGE('',*,*,#2731,.F.);
#3512=ORIENTED_EDGE('',*,*,#2732,.T.);
#3513=ORIENTED_EDGE('',*,*,#2730,.F.);
#3514=ORIENTED_EDGE('',*,*,#2733,.F.);
#3515=ORIENTED_EDGE('',*,*,#2734,.F.);
#3516=ORIENTED_EDGE('',*,*,#2735,.F.);
#3517=ORIENTED_EDGE('',*,*,#2734,.T.);
#3518=ORIENTED_EDGE('',*,*,#2736,.F.);
#3519=ORIENTED_EDGE('',*,*,#2737,.F.);
#3520=ORIENTED_EDGE('',*,*,#2738,.F.);
#3521=ORIENTED_EDGE('',*,*,#2737,.T.);
#3522=ORIENTED_EDGE('',*,*,#2739,.F.);
#3523=ORIENTED_EDGE('',*,*,#2614,.F.);
#3524=ORIENTED_EDGE('',*,*,#2740,.F.);
#3525=ORIENTED_EDGE('',*,*,#2741,.F.);
#3526=ORIENTED_EDGE('',*,*,#2742,.F.);
#3527=ORIENTED_EDGE('',*,*,#2743,.F.);
#3528=ORIENTED_EDGE('',*,*,#2744,.F.);
#3529=ORIENTED_EDGE('',*,*,#2745,.F.);
#3530=ORIENTED_EDGE('',*,*,#2746,.F.);
#3531=ORIENTED_EDGE('',*,*,#2747,.F.);
#3532=ORIENTED_EDGE('',*,*,#2741,.T.);
#3533=ORIENTED_EDGE('',*,*,#2748,.F.);
#3534=ORIENTED_EDGE('',*,*,#2749,.T.);
#3535=ORIENTED_EDGE('',*,*,#2750,.F.);
#3536=ORIENTED_EDGE('',*,*,#2747,.T.);
#3537=ORIENTED_EDGE('',*,*,#2751,.F.);
#3538=ORIENTED_EDGE('',*,*,#2752,.T.);
#3539=ORIENTED_EDGE('',*,*,#2753,.F.);
#3540=ORIENTED_EDGE('',*,*,#2743,.T.);
#3541=ORIENTED_EDGE('',*,*,#2754,.F.);
#3542=ORIENTED_EDGE('',*,*,#2755,.T.);
#3543=ORIENTED_EDGE('',*,*,#2756,.F.);
#3544=ORIENTED_EDGE('',*,*,#2745,.T.);
#3545=ORIENTED_EDGE('',*,*,#2757,.F.);
#3546=ORIENTED_EDGE('',*,*,#2758,.T.);
#3547=ORIENTED_EDGE('',*,*,#2759,.F.);
#3548=ORIENTED_EDGE('',*,*,#2760,.F.);
#3549=ORIENTED_EDGE('',*,*,#2752,.F.);
#3550=ORIENTED_EDGE('',*,*,#2761,.F.);
#3551=ORIENTED_EDGE('',*,*,#2758,.F.);
#3552=ORIENTED_EDGE('',*,*,#2762,.F.);
#3553=ORIENTED_EDGE('',*,*,#2763,.F.);
#3554=ORIENTED_EDGE('',*,*,#2764,.F.);
#3555=ORIENTED_EDGE('',*,*,#2765,.F.);
#3556=ORIENTED_EDGE('',*,*,#2765,.T.);
#3557=ORIENTED_EDGE('',*,*,#2766,.F.);
#3558=ORIENTED_EDGE('',*,*,#2767,.T.);
#3559=ORIENTED_EDGE('',*,*,#2768,.F.);
#3560=ORIENTED_EDGE('',*,*,#2763,.T.);
#3561=ORIENTED_EDGE('',*,*,#2769,.F.);
#3562=ORIENTED_EDGE('',*,*,#2770,.T.);
#3563=ORIENTED_EDGE('',*,*,#2771,.F.);
#3564=ORIENTED_EDGE('',*,*,#2772,.F.);
#3565=ORIENTED_EDGE('',*,*,#2773,.F.);
#3566=ORIENTED_EDGE('',*,*,#2774,.F.);
#3567=ORIENTED_EDGE('',*,*,#2775,.F.);
#3568=ORIENTED_EDGE('',*,*,#2776,.F.);
#3569=ORIENTED_EDGE('',*,*,#2777,.F.);
#3570=ORIENTED_EDGE('',*,*,#2778,.F.);
#3571=ORIENTED_EDGE('',*,*,#2779,.F.);
#3572=ORIENTED_EDGE('',*,*,#2773,.T.);
#3573=ORIENTED_EDGE('',*,*,#2780,.F.);
#3574=ORIENTED_EDGE('',*,*,#2781,.T.);
#3575=ORIENTED_EDGE('',*,*,#2782,.F.);
#3576=ORIENTED_EDGE('',*,*,#2779,.T.);
#3577=ORIENTED_EDGE('',*,*,#2783,.F.);
#3578=ORIENTED_EDGE('',*,*,#2784,.T.);
#3579=ORIENTED_EDGE('',*,*,#2785,.F.);
#3580=ORIENTED_EDGE('',*,*,#2775,.T.);
#3581=ORIENTED_EDGE('',*,*,#2786,.F.);
#3582=ORIENTED_EDGE('',*,*,#2787,.T.);
#3583=ORIENTED_EDGE('',*,*,#2788,.F.);
#3584=ORIENTED_EDGE('',*,*,#2777,.T.);
#3585=ORIENTED_EDGE('',*,*,#2789,.F.);
#3586=ORIENTED_EDGE('',*,*,#2790,.T.);
#3587=ORIENTED_EDGE('',*,*,#2791,.F.);
#3588=ORIENTED_EDGE('',*,*,#2792,.F.);
#3589=ORIENTED_EDGE('',*,*,#2793,.F.);
#3590=ORIENTED_EDGE('',*,*,#2794,.F.);
#3591=ORIENTED_EDGE('',*,*,#2795,.F.);
#3592=ORIENTED_EDGE('',*,*,#2796,.F.);
#3593=ORIENTED_EDGE('',*,*,#2797,.F.);
#3594=ORIENTED_EDGE('',*,*,#2798,.F.);
#3595=ORIENTED_EDGE('',*,*,#2799,.F.);
#3596=ORIENTED_EDGE('',*,*,#2793,.T.);
#3597=ORIENTED_EDGE('',*,*,#2800,.F.);
#3598=ORIENTED_EDGE('',*,*,#2801,.T.);
#3599=ORIENTED_EDGE('',*,*,#2802,.F.);
#3600=ORIENTED_EDGE('',*,*,#2799,.T.);
#3601=ORIENTED_EDGE('',*,*,#2803,.F.);
#3602=ORIENTED_EDGE('',*,*,#2804,.T.);
#3603=ORIENTED_EDGE('',*,*,#2805,.F.);
#3604=ORIENTED_EDGE('',*,*,#2795,.T.);
#3605=ORIENTED_EDGE('',*,*,#2806,.F.);
#3606=ORIENTED_EDGE('',*,*,#2807,.T.);
#3607=ORIENTED_EDGE('',*,*,#2808,.F.);
#3608=ORIENTED_EDGE('',*,*,#2797,.T.);
#3609=ORIENTED_EDGE('',*,*,#2809,.F.);
#3610=ORIENTED_EDGE('',*,*,#2810,.T.);
#3611=ORIENTED_EDGE('',*,*,#2811,.F.);
#3612=ORIENTED_EDGE('',*,*,#2812,.F.);
#3613=ORIENTED_EDGE('',*,*,#2767,.F.);
#3614=ORIENTED_EDGE('',*,*,#2813,.F.);
#3615=ORIENTED_EDGE('',*,*,#2770,.F.);
#3616=ORIENTED_EDGE('',*,*,#2814,.F.);
#3617=ORIENTED_EDGE('',*,*,#2815,.F.);
#3618=ORIENTED_EDGE('',*,*,#2816,.F.);
#3619=ORIENTED_EDGE('',*,*,#2817,.F.);
#3620=ORIENTED_EDGE('',*,*,#2817,.T.);
#3621=ORIENTED_EDGE('',*,*,#2818,.F.);
#3622=ORIENTED_EDGE('',*,*,#2819,.T.);
#3623=ORIENTED_EDGE('',*,*,#2820,.F.);
#3624=ORIENTED_EDGE('',*,*,#2815,.T.);
#3625=ORIENTED_EDGE('',*,*,#2821,.F.);
#3626=ORIENTED_EDGE('',*,*,#2822,.T.);
#3627=ORIENTED_EDGE('',*,*,#2823,.F.);
#3628=ORIENTED_EDGE('',*,*,#2824,.F.);
#3629=ORIENTED_EDGE('',*,*,#2804,.F.);
#3630=ORIENTED_EDGE('',*,*,#2825,.F.);
#3631=ORIENTED_EDGE('',*,*,#2810,.F.);
#3632=ORIENTED_EDGE('',*,*,#2826,.F.);
#3633=ORIENTED_EDGE('',*,*,#2787,.F.);
#3634=ORIENTED_EDGE('',*,*,#2827,.F.);
#3635=ORIENTED_EDGE('',*,*,#2781,.F.);
#3636=ORIENTED_EDGE('',*,*,#2828,.F.);
#3637=ORIENTED_EDGE('',*,*,#2819,.F.);
#3638=ORIENTED_EDGE('',*,*,#2829,.F.);
#3639=ORIENTED_EDGE('',*,*,#2822,.F.);
#3640=ORIENTED_EDGE('',*,*,#2830,.F.);
#3641=ORIENTED_EDGE('',*,*,#2831,.F.);
#3642=ORIENTED_EDGE('',*,*,#2832,.F.);
#3643=ORIENTED_EDGE('',*,*,#2833,.F.);
#3644=ORIENTED_EDGE('',*,*,#2833,.T.);
#3645=ORIENTED_EDGE('',*,*,#2834,.F.);
#3646=ORIENTED_EDGE('',*,*,#2835,.T.);
#3647=ORIENTED_EDGE('',*,*,#2836,.F.);
#3648=ORIENTED_EDGE('',*,*,#2831,.T.);
#3649=ORIENTED_EDGE('',*,*,#2837,.F.);
#3650=ORIENTED_EDGE('',*,*,#2838,.T.);
#3651=ORIENTED_EDGE('',*,*,#2839,.F.);
#3652=ORIENTED_EDGE('',*,*,#2840,.F.);
#3653=ORIENTED_EDGE('',*,*,#2784,.F.);
#3654=ORIENTED_EDGE('',*,*,#2841,.F.);
#3655=ORIENTED_EDGE('',*,*,#2790,.F.);
#3656=ORIENTED_EDGE('',*,*,#2842,.F.);
#3657=ORIENTED_EDGE('',*,*,#2755,.F.);
#3658=ORIENTED_EDGE('',*,*,#2843,.F.);
#3659=ORIENTED_EDGE('',*,*,#2749,.F.);
#3660=ORIENTED_EDGE('',*,*,#2844,.T.);
#3661=ORIENTED_EDGE('',*,*,#2845,.F.);
#3662=ORIENTED_EDGE('',*,*,#2846,.F.);
#3663=ORIENTED_EDGE('',*,*,#2847,.F.);
#3664=ORIENTED_EDGE('',*,*,#2848,.F.);
#3665=ORIENTED_EDGE('',*,*,#2847,.T.);
#3666=ORIENTED_EDGE('',*,*,#2849,.F.);
#3667=ORIENTED_EDGE('',*,*,#2850,.F.);
#3668=ORIENTED_EDGE('',*,*,#2851,.F.);
#3669=ORIENTED_EDGE('',*,*,#2850,.T.);
#3670=ORIENTED_EDGE('',*,*,#2852,.F.);
#3671=ORIENTED_EDGE('',*,*,#2853,.F.);
#3672=ORIENTED_EDGE('',*,*,#2845,.T.);
#3673=ORIENTED_EDGE('',*,*,#2854,.F.);
#3674=ORIENTED_EDGE('',*,*,#2855,.T.);
#3675=ORIENTED_EDGE('',*,*,#2856,.F.);
#3676=ORIENTED_EDGE('',*,*,#2853,.T.);
#3677=ORIENTED_EDGE('',*,*,#2857,.F.);
#3678=ORIENTED_EDGE('',*,*,#2858,.T.);
#3679=ORIENTED_EDGE('',*,*,#2859,.F.);
#3680=ORIENTED_EDGE('',*,*,#2860,.T.);
#3681=ORIENTED_EDGE('',*,*,#2858,.F.);
#3682=ORIENTED_EDGE('',*,*,#2861,.F.);
#3683=ORIENTED_EDGE('',*,*,#2862,.F.);
#3684=ORIENTED_EDGE('',*,*,#2863,.F.);
#3685=ORIENTED_EDGE('',*,*,#2862,.T.);
#3686=ORIENTED_EDGE('',*,*,#2864,.F.);
#3687=ORIENTED_EDGE('',*,*,#2865,.F.);
#3688=ORIENTED_EDGE('',*,*,#2866,.F.);
#3689=ORIENTED_EDGE('',*,*,#2865,.T.);
#3690=ORIENTED_EDGE('',*,*,#2867,.F.);
#3691=ORIENTED_EDGE('',*,*,#2868,.F.);
#3692=ORIENTED_EDGE('',*,*,#2868,.T.);
#3693=ORIENTED_EDGE('',*,*,#2869,.F.);
#3694=ORIENTED_EDGE('',*,*,#2870,.T.);
#3695=ORIENTED_EDGE('',*,*,#2871,.F.);
#3696=ORIENTED_EDGE('',*,*,#2872,.T.);
#3697=ORIENTED_EDGE('',*,*,#2873,.F.);
#3698=ORIENTED_EDGE('',*,*,#2874,.F.);
#3699=ORIENTED_EDGE('',*,*,#2875,.F.);
#3700=ORIENTED_EDGE('',*,*,#2876,.F.);
#3701=ORIENTED_EDGE('',*,*,#2875,.T.);
#3702=ORIENTED_EDGE('',*,*,#2877,.F.);
#3703=ORIENTED_EDGE('',*,*,#2878,.F.);
#3704=ORIENTED_EDGE('',*,*,#2879,.F.);
#3705=ORIENTED_EDGE('',*,*,#2878,.T.);
#3706=ORIENTED_EDGE('',*,*,#2880,.F.);
#3707=ORIENTED_EDGE('',*,*,#2881,.F.);
#3708=ORIENTED_EDGE('',*,*,#2873,.T.);
#3709=ORIENTED_EDGE('',*,*,#2882,.F.);
#3710=ORIENTED_EDGE('',*,*,#2883,.T.);
#3711=ORIENTED_EDGE('',*,*,#2884,.F.);
#3712=ORIENTED_EDGE('',*,*,#2881,.T.);
#3713=ORIENTED_EDGE('',*,*,#2885,.F.);
#3714=ORIENTED_EDGE('',*,*,#2886,.T.);
#3715=ORIENTED_EDGE('',*,*,#2887,.F.);
#3716=ORIENTED_EDGE('',*,*,#2888,.T.);
#3717=ORIENTED_EDGE('',*,*,#2889,.F.);
#3718=ORIENTED_EDGE('',*,*,#2890,.F.);
#3719=ORIENTED_EDGE('',*,*,#2891,.F.);
#3720=ORIENTED_EDGE('',*,*,#2892,.F.);
#3721=ORIENTED_EDGE('',*,*,#2891,.T.);
#3722=ORIENTED_EDGE('',*,*,#2893,.F.);
#3723=ORIENTED_EDGE('',*,*,#2894,.F.);
#3724=ORIENTED_EDGE('',*,*,#2895,.F.);
#3725=ORIENTED_EDGE('',*,*,#2894,.T.);
#3726=ORIENTED_EDGE('',*,*,#2896,.F.);
#3727=ORIENTED_EDGE('',*,*,#2897,.F.);
#3728=ORIENTED_EDGE('',*,*,#2889,.T.);
#3729=ORIENTED_EDGE('',*,*,#2898,.F.);
#3730=ORIENTED_EDGE('',*,*,#2899,.T.);
#3731=ORIENTED_EDGE('',*,*,#2900,.F.);
#3732=ORIENTED_EDGE('',*,*,#2897,.T.);
#3733=ORIENTED_EDGE('',*,*,#2901,.F.);
#3734=ORIENTED_EDGE('',*,*,#2902,.T.);
#3735=ORIENTED_EDGE('',*,*,#2903,.F.);
#3736=ORIENTED_EDGE('',*,*,#2904,.T.);
#3737=ORIENTED_EDGE('',*,*,#2886,.F.);
#3738=ORIENTED_EDGE('',*,*,#2905,.F.);
#3739=ORIENTED_EDGE('',*,*,#2906,.F.);
#3740=ORIENTED_EDGE('',*,*,#2907,.F.);
#3741=ORIENTED_EDGE('',*,*,#2906,.T.);
#3742=ORIENTED_EDGE('',*,*,#2908,.F.);
#3743=ORIENTED_EDGE('',*,*,#2909,.F.);
#3744=ORIENTED_EDGE('',*,*,#2910,.F.);
#3745=ORIENTED_EDGE('',*,*,#2909,.T.);
#3746=ORIENTED_EDGE('',*,*,#2911,.F.);
#3747=ORIENTED_EDGE('',*,*,#2899,.F.);
#3748=ORIENTED_EDGE('',*,*,#2912,.T.);
#3749=ORIENTED_EDGE('',*,*,#2582,.F.);
#3750=ORIENTED_EDGE('',*,*,#2913,.F.);
#3751=ORIENTED_EDGE('',*,*,#2914,.F.);
#3752=ORIENTED_EDGE('',*,*,#2915,.F.);
#3753=ORIENTED_EDGE('',*,*,#2914,.T.);
#3754=ORIENTED_EDGE('',*,*,#2916,.F.);
#3755=ORIENTED_EDGE('',*,*,#2917,.F.);
#3756=ORIENTED_EDGE('',*,*,#2918,.F.);
#3757=ORIENTED_EDGE('',*,*,#2917,.T.);
#3758=ORIENTED_EDGE('',*,*,#2919,.F.);
#3759=ORIENTED_EDGE('',*,*,#2855,.F.);
#3760=ORIENTED_EDGE('',*,*,#2920,.T.);
#3761=ORIENTED_EDGE('',*,*,#2870,.F.);
#3762=ORIENTED_EDGE('',*,*,#2921,.F.);
#3763=ORIENTED_EDGE('',*,*,#2922,.F.);
#3764=ORIENTED_EDGE('',*,*,#2923,.F.);
#3765=ORIENTED_EDGE('',*,*,#2922,.T.);
#3766=ORIENTED_EDGE('',*,*,#2924,.F.);
#3767=ORIENTED_EDGE('',*,*,#2925,.F.);
#3768=ORIENTED_EDGE('',*,*,#2926,.F.);
#3769=ORIENTED_EDGE('',*,*,#2925,.T.);
#3770=ORIENTED_EDGE('',*,*,#2927,.F.);
#3771=ORIENTED_EDGE('',*,*,#2883,.F.);
#3772=ORIENTED_EDGE('',*,*,#2928,.T.);
#3773=ORIENTED_EDGE('',*,*,#2902,.F.);
#3774=ORIENTED_EDGE('',*,*,#2929,.F.);
#3775=ORIENTED_EDGE('',*,*,#2930,.F.);
#3776=ORIENTED_EDGE('',*,*,#2931,.F.);
#3777=ORIENTED_EDGE('',*,*,#2930,.T.);
#3778=ORIENTED_EDGE('',*,*,#2932,.F.);
#3779=ORIENTED_EDGE('',*,*,#2933,.F.);
#3780=ORIENTED_EDGE('',*,*,#2934,.F.);
#3781=ORIENTED_EDGE('',*,*,#2933,.T.);
#3782=ORIENTED_EDGE('',*,*,#2935,.F.);
#3783=ORIENTED_EDGE('',*,*,#2936,.F.);
#3784=ORIENTED_EDGE('',*,*,#2936,.T.);
#3785=ORIENTED_EDGE('',*,*,#2937,.F.);
#3786=ORIENTED_EDGE('',*,*,#2938,.T.);
#3787=ORIENTED_EDGE('',*,*,#2939,.F.);
#3788=ORIENTED_EDGE('',*,*,#2940,.F.);
#3789=ORIENTED_EDGE('',*,*,#2835,.F.);
#3790=ORIENTED_EDGE('',*,*,#2941,.F.);
#3791=ORIENTED_EDGE('',*,*,#2838,.F.);
#3792=ORIENTED_EDGE('',*,*,#2942,.F.);
#3793=ORIENTED_EDGE('',*,*,#2943,.F.);
#3794=ORIENTED_EDGE('',*,*,#2944,.F.);
#3795=ORIENTED_EDGE('',*,*,#2945,.F.);
#3796=ORIENTED_EDGE('',*,*,#2945,.T.);
#3797=ORIENTED_EDGE('',*,*,#2946,.F.);
#3798=ORIENTED_EDGE('',*,*,#2947,.T.);
#3799=ORIENTED_EDGE('',*,*,#2948,.F.);
#3800=ORIENTED_EDGE('',*,*,#2943,.T.);
#3801=ORIENTED_EDGE('',*,*,#2949,.F.);
#3802=ORIENTED_EDGE('',*,*,#2950,.T.);
#3803=ORIENTED_EDGE('',*,*,#2951,.F.);
#3804=ORIENTED_EDGE('',*,*,#2952,.F.);
#3805=ORIENTED_EDGE('',*,*,#2953,.F.);
#3806=ORIENTED_EDGE('',*,*,#2954,.F.);
#3807=ORIENTED_EDGE('',*,*,#2955,.F.);
#3808=ORIENTED_EDGE('',*,*,#2956,.F.);
#3809=ORIENTED_EDGE('',*,*,#2666,.F.);
#3810=ORIENTED_EDGE('',*,*,#2957,.F.);
#3811=ORIENTED_EDGE('',*,*,#2663,.F.);
#3812=ORIENTED_EDGE('',*,*,#2953,.T.);
#3813=ORIENTED_EDGE('',*,*,#2958,.F.);
#3814=ORIENTED_EDGE('',*,*,#2959,.T.);
#3815=ORIENTED_EDGE('',*,*,#2960,.F.);
#3816=ORIENTED_EDGE('',*,*,#2955,.T.);
#3817=ORIENTED_EDGE('',*,*,#2961,.F.);
#3818=ORIENTED_EDGE('',*,*,#2962,.T.);
#3819=ORIENTED_EDGE('',*,*,#2963,.F.);
#3820=ORIENTED_EDGE('',*,*,#2964,.F.);
#3821=ORIENTED_EDGE('',*,*,#2947,.F.);
#3822=ORIENTED_EDGE('',*,*,#2965,.F.);
#3823=ORIENTED_EDGE('',*,*,#2950,.F.);
#3824=ORIENTED_EDGE('',*,*,#2966,.F.);
#3825=ORIENTED_EDGE('',*,*,#2962,.F.);
#3826=ORIENTED_EDGE('',*,*,#2967,.F.);
#3827=ORIENTED_EDGE('',*,*,#2959,.F.);
#3828=ORIENTED_EDGE('',*,*,#2968,.T.);
#3829=ORIENTED_EDGE('',*,*,#2969,.F.);
#3830=ORIENTED_EDGE('',*,*,#2970,.F.);
#3831=ORIENTED_EDGE('',*,*,#2971,.F.);
#3832=ORIENTED_EDGE('',*,*,#2972,.F.);
#3833=ORIENTED_EDGE('',*,*,#2971,.T.);
#3834=ORIENTED_EDGE('',*,*,#2973,.F.);
#3835=ORIENTED_EDGE('',*,*,#2974,.F.);
#3836=ORIENTED_EDGE('',*,*,#2975,.F.);
#3837=ORIENTED_EDGE('',*,*,#2974,.T.);
#3838=ORIENTED_EDGE('',*,*,#2976,.F.);
#3839=ORIENTED_EDGE('',*,*,#2977,.F.);
#3840=ORIENTED_EDGE('',*,*,#2969,.T.);
#3841=ORIENTED_EDGE('',*,*,#2978,.F.);
#3842=ORIENTED_EDGE('',*,*,#2979,.T.);
#3843=ORIENTED_EDGE('',*,*,#2980,.F.);
#3844=ORIENTED_EDGE('',*,*,#2977,.T.);
#3845=ORIENTED_EDGE('',*,*,#2981,.F.);
#3846=ORIENTED_EDGE('',*,*,#2982,.T.);
#3847=ORIENTED_EDGE('',*,*,#2983,.F.);
#3848=ORIENTED_EDGE('',*,*,#2984,.T.);
#3849=ORIENTED_EDGE('',*,*,#2982,.F.);
#3850=ORIENTED_EDGE('',*,*,#2985,.F.);
#3851=ORIENTED_EDGE('',*,*,#2986,.F.);
#3852=ORIENTED_EDGE('',*,*,#2987,.F.);
#3853=ORIENTED_EDGE('',*,*,#2986,.T.);
#3854=ORIENTED_EDGE('',*,*,#2988,.F.);
#3855=ORIENTED_EDGE('',*,*,#2989,.F.);
#3856=ORIENTED_EDGE('',*,*,#2990,.F.);
#3857=ORIENTED_EDGE('',*,*,#2989,.T.);
#3858=ORIENTED_EDGE('',*,*,#2991,.F.);
#3859=ORIENTED_EDGE('',*,*,#2992,.F.);
#3860=ORIENTED_EDGE('',*,*,#2992,.T.);
#3861=ORIENTED_EDGE('',*,*,#2993,.F.);
#3862=ORIENTED_EDGE('',*,*,#2994,.T.);
#3863=ORIENTED_EDGE('',*,*,#2995,.F.);
#3864=ORIENTED_EDGE('',*,*,#2996,.T.);
#3865=ORIENTED_EDGE('',*,*,#2997,.F.);
#3866=ORIENTED_EDGE('',*,*,#2998,.F.);
#3867=ORIENTED_EDGE('',*,*,#2999,.F.);
#3868=ORIENTED_EDGE('',*,*,#3000,.F.);
#3869=ORIENTED_EDGE('',*,*,#2999,.T.);
#3870=ORIENTED_EDGE('',*,*,#3001,.F.);
#3871=ORIENTED_EDGE('',*,*,#3002,.F.);
#3872=ORIENTED_EDGE('',*,*,#3003,.F.);
#3873=ORIENTED_EDGE('',*,*,#3002,.T.);
#3874=ORIENTED_EDGE('',*,*,#3004,.F.);
#3875=ORIENTED_EDGE('',*,*,#3005,.F.);
#3876=ORIENTED_EDGE('',*,*,#2997,.T.);
#3877=ORIENTED_EDGE('',*,*,#3006,.F.);
#3878=ORIENTED_EDGE('',*,*,#3007,.T.);
#3879=ORIENTED_EDGE('',*,*,#3008,.F.);
#3880=ORIENTED_EDGE('',*,*,#3005,.T.);
#3881=ORIENTED_EDGE('',*,*,#3009,.F.);
#3882=ORIENTED_EDGE('',*,*,#3010,.T.);
#3883=ORIENTED_EDGE('',*,*,#3011,.F.);
#3884=ORIENTED_EDGE('',*,*,#3012,.T.);
#3885=ORIENTED_EDGE('',*,*,#2994,.F.);
#3886=ORIENTED_EDGE('',*,*,#3013,.F.);
#3887=ORIENTED_EDGE('',*,*,#3014,.F.);
#3888=ORIENTED_EDGE('',*,*,#3015,.F.);
#3889=ORIENTED_EDGE('',*,*,#3014,.T.);
#3890=ORIENTED_EDGE('',*,*,#3016,.F.);
#3891=ORIENTED_EDGE('',*,*,#3017,.F.);
#3892=ORIENTED_EDGE('',*,*,#3018,.F.);
#3893=ORIENTED_EDGE('',*,*,#3017,.T.);
#3894=ORIENTED_EDGE('',*,*,#3019,.F.);
#3895=ORIENTED_EDGE('',*,*,#3020,.F.);
#3896=ORIENTED_EDGE('',*,*,#3020,.T.);
#3897=ORIENTED_EDGE('',*,*,#3021,.F.);
#3898=ORIENTED_EDGE('',*,*,#3022,.T.);
#3899=ORIENTED_EDGE('',*,*,#3023,.F.);
#3900=ORIENTED_EDGE('',*,*,#3024,.T.);
#3901=ORIENTED_EDGE('',*,*,#2938,.F.);
#3902=ORIENTED_EDGE('',*,*,#3025,.F.);
#3903=ORIENTED_EDGE('',*,*,#3026,.F.);
#3904=ORIENTED_EDGE('',*,*,#3027,.F.);
#3905=ORIENTED_EDGE('',*,*,#3026,.T.);
#3906=ORIENTED_EDGE('',*,*,#3028,.F.);
#3907=ORIENTED_EDGE('',*,*,#3029,.F.);
#3908=ORIENTED_EDGE('',*,*,#3030,.F.);
#3909=ORIENTED_EDGE('',*,*,#3029,.T.);
#3910=ORIENTED_EDGE('',*,*,#3031,.F.);
#3911=ORIENTED_EDGE('',*,*,#3032,.F.);
#3912=ORIENTED_EDGE('',*,*,#3032,.T.);
#3913=ORIENTED_EDGE('',*,*,#3033,.F.);
#3914=ORIENTED_EDGE('',*,*,#3034,.T.);
#3915=ORIENTED_EDGE('',*,*,#3035,.F.);
#3916=ORIENTED_EDGE('',*,*,#3036,.T.);
#3917=ORIENTED_EDGE('',*,*,#3010,.F.);
#3918=ORIENTED_EDGE('',*,*,#3037,.F.);
#3919=ORIENTED_EDGE('',*,*,#3038,.F.);
#3920=ORIENTED_EDGE('',*,*,#3039,.F.);
#3921=ORIENTED_EDGE('',*,*,#3038,.T.);
#3922=ORIENTED_EDGE('',*,*,#3040,.F.);
#3923=ORIENTED_EDGE('',*,*,#3041,.F.);
#3924=ORIENTED_EDGE('',*,*,#3042,.F.);
#3925=ORIENTED_EDGE('',*,*,#3041,.T.);
#3926=ORIENTED_EDGE('',*,*,#3043,.F.);
#3927=ORIENTED_EDGE('',*,*,#2695,.F.);
#3928=ORIENTED_EDGE('',*,*,#3044,.T.);
#3929=ORIENTED_EDGE('',*,*,#3022,.F.);
#3930=ORIENTED_EDGE('',*,*,#3045,.F.);
#3931=ORIENTED_EDGE('',*,*,#3046,.F.);
#3932=ORIENTED_EDGE('',*,*,#3047,.F.);
#3933=ORIENTED_EDGE('',*,*,#3046,.T.);
#3934=ORIENTED_EDGE('',*,*,#3048,.F.);
#3935=ORIENTED_EDGE('',*,*,#3049,.F.);
#3936=ORIENTED_EDGE('',*,*,#3050,.F.);
#3937=ORIENTED_EDGE('',*,*,#3049,.T.);
#3938=ORIENTED_EDGE('',*,*,#3051,.F.);
#3939=ORIENTED_EDGE('',*,*,#3007,.F.);
#3940=ORIENTED_EDGE('',*,*,#3052,.T.);
#3941=ORIENTED_EDGE('',*,*,#3034,.F.);
#3942=ORIENTED_EDGE('',*,*,#3053,.F.);
#3943=ORIENTED_EDGE('',*,*,#3054,.F.);
#3944=ORIENTED_EDGE('',*,*,#3055,.F.);
#3945=ORIENTED_EDGE('',*,*,#3054,.T.);
#3946=ORIENTED_EDGE('',*,*,#3056,.F.);
#3947=ORIENTED_EDGE('',*,*,#3057,.F.);
#3948=ORIENTED_EDGE('',*,*,#3058,.F.);
#3949=ORIENTED_EDGE('',*,*,#3057,.T.);
#3950=ORIENTED_EDGE('',*,*,#3059,.F.);
#3951=ORIENTED_EDGE('',*,*,#2979,.F.);
#3952=ORIENTED_EDGE('',*,*,#3060,.F.);
#3953=ORIENTED_EDGE('',*,*,#2651,.F.);
#3954=ORIENTED_EDGE('',*,*,#3061,.F.);
#3955=ORIENTED_EDGE('',*,*,#2654,.F.);
#3956=ORIENTED_EDGE('',*,*,#3062,.F.);
#3957=ORIENTED_EDGE('',*,*,#2807,.F.);
#3958=ORIENTED_EDGE('',*,*,#3063,.F.);
#3959=ORIENTED_EDGE('',*,*,#2801,.F.);
#3960=ORIENTED_EDGE('',*,*,#3064,.F.);
#3961=ORIENTED_EDGE('',*,*,#3065,.T.);
#3962=ORIENTED_EDGE('',*,*,#3066,.F.);
#3963=ORIENTED_EDGE('',*,*,#3065,.F.);
#3964=ORIENTED_EDGE('',*,*,#2978,.T.);
#3965=ORIENTED_EDGE('',*,*,#2968,.F.);
#3966=ORIENTED_EDGE('',*,*,#2972,.T.);
#3967=ORIENTED_EDGE('',*,*,#2975,.T.);
#3968=ORIENTED_EDGE('',*,*,#2983,.T.);
#3969=ORIENTED_EDGE('',*,*,#2984,.F.);
#3970=ORIENTED_EDGE('',*,*,#2987,.T.);
#3971=ORIENTED_EDGE('',*,*,#2990,.T.);
#3972=ORIENTED_EDGE('',*,*,#2995,.T.);
#3973=ORIENTED_EDGE('',*,*,#3012,.F.);
#3974=ORIENTED_EDGE('',*,*,#3015,.T.);
#3975=ORIENTED_EDGE('',*,*,#3018,.T.);
#3976=ORIENTED_EDGE('',*,*,#3023,.T.);
#3977=ORIENTED_EDGE('',*,*,#3044,.F.);
#3978=ORIENTED_EDGE('',*,*,#3047,.T.);
#3979=ORIENTED_EDGE('',*,*,#3050,.T.);
#3980=ORIENTED_EDGE('',*,*,#3006,.T.);
#3981=ORIENTED_EDGE('',*,*,#2996,.F.);
#3982=ORIENTED_EDGE('',*,*,#3000,.T.);
#3983=ORIENTED_EDGE('',*,*,#3003,.T.);
#3984=ORIENTED_EDGE('',*,*,#3011,.T.);
#3985=ORIENTED_EDGE('',*,*,#3036,.F.);
#3986=ORIENTED_EDGE('',*,*,#3039,.T.);
#3987=ORIENTED_EDGE('',*,*,#3042,.T.);
#3988=ORIENTED_EDGE('',*,*,#2694,.T.);
#3989=ORIENTED_EDGE('',*,*,#2684,.F.);
#3990=ORIENTED_EDGE('',*,*,#2688,.T.);
#3991=ORIENTED_EDGE('',*,*,#2691,.T.);
#3992=ORIENTED_EDGE('',*,*,#2699,.T.);
#3993=ORIENTED_EDGE('',*,*,#2700,.F.);
#3994=ORIENTED_EDGE('',*,*,#2703,.T.);
#3995=ORIENTED_EDGE('',*,*,#2706,.T.);
#3996=ORIENTED_EDGE('',*,*,#2711,.T.);
#3997=ORIENTED_EDGE('',*,*,#2712,.F.);
#3998=ORIENTED_EDGE('',*,*,#2715,.T.);
#3999=ORIENTED_EDGE('',*,*,#2718,.T.);
#4000=ORIENTED_EDGE('',*,*,#2678,.T.);
#4001=ORIENTED_EDGE('',*,*,#2668,.F.);
#4002=ORIENTED_EDGE('',*,*,#2672,.T.);
#4003=ORIENTED_EDGE('',*,*,#2675,.T.);
#4004=ORIENTED_EDGE('',*,*,#2683,.T.);
#4005=ORIENTED_EDGE('',*,*,#2720,.F.);
#4006=ORIENTED_EDGE('',*,*,#2723,.T.);
#4007=ORIENTED_EDGE('',*,*,#2726,.T.);
#4008=ORIENTED_EDGE('',*,*,#2731,.T.);
#4009=ORIENTED_EDGE('',*,*,#2732,.F.);
#4010=ORIENTED_EDGE('',*,*,#2735,.T.);
#4011=ORIENTED_EDGE('',*,*,#2738,.T.);
#4012=ORIENTED_EDGE('',*,*,#2613,.T.);
#4013=ORIENTED_EDGE('',*,*,#2604,.F.);
#4014=ORIENTED_EDGE('',*,*,#2608,.T.);
#4015=ORIENTED_EDGE('',*,*,#2611,.T.);
#4016=ORIENTED_EDGE('',*,*,#2534,.T.);
#4017=ORIENTED_EDGE('',*,*,#2524,.F.);
#4018=ORIENTED_EDGE('',*,*,#2528,.T.);
#4019=ORIENTED_EDGE('',*,*,#2531,.T.);
#4020=ORIENTED_EDGE('',*,*,#2539,.T.);
#4021=ORIENTED_EDGE('',*,*,#2556,.F.);
#4022=ORIENTED_EDGE('',*,*,#2559,.T.);
#4023=ORIENTED_EDGE('',*,*,#2562,.T.);
#4024=ORIENTED_EDGE('',*,*,#2567,.T.);
#4025=ORIENTED_EDGE('',*,*,#2584,.F.);
#4026=ORIENTED_EDGE('',*,*,#2587,.T.);
#4027=ORIENTED_EDGE('',*,*,#2590,.T.);
#4028=ORIENTED_EDGE('',*,*,#2550,.T.);
#4029=ORIENTED_EDGE('',*,*,#2540,.F.);
#4030=ORIENTED_EDGE('',*,*,#2544,.T.);
#4031=ORIENTED_EDGE('',*,*,#2547,.T.);
#4032=ORIENTED_EDGE('',*,*,#2555,.T.);
#4033=ORIENTED_EDGE('',*,*,#2592,.F.);
#4034=ORIENTED_EDGE('',*,*,#2595,.T.);
#4035=ORIENTED_EDGE('',*,*,#2598,.T.);
#4036=ORIENTED_EDGE('',*,*,#2603,.T.);
#4037=ORIENTED_EDGE('',*,*,#2616,.F.);
#4038=ORIENTED_EDGE('',*,*,#2619,.T.);
#4039=ORIENTED_EDGE('',*,*,#2622,.T.);
#4040=ORIENTED_EDGE('',*,*,#2578,.T.);
#4041=ORIENTED_EDGE('',*,*,#2568,.F.);
#4042=ORIENTED_EDGE('',*,*,#2572,.T.);
#4043=ORIENTED_EDGE('',*,*,#2575,.T.);
#4044=ORIENTED_EDGE('',*,*,#2583,.T.);
#4045=ORIENTED_EDGE('',*,*,#2912,.F.);
#4046=ORIENTED_EDGE('',*,*,#2915,.T.);
#4047=ORIENTED_EDGE('',*,*,#2918,.T.);
#4048=ORIENTED_EDGE('',*,*,#2854,.T.);
#4049=ORIENTED_EDGE('',*,*,#2844,.F.);
#4050=ORIENTED_EDGE('',*,*,#2848,.T.);
#4051=ORIENTED_EDGE('',*,*,#2851,.T.);
#4052=ORIENTED_EDGE('',*,*,#2859,.T.);
#4053=ORIENTED_EDGE('',*,*,#2860,.F.);
#4054=ORIENTED_EDGE('',*,*,#2863,.T.);
#4055=ORIENTED_EDGE('',*,*,#2866,.T.);
#4056=ORIENTED_EDGE('',*,*,#2871,.T.);
#4057=ORIENTED_EDGE('',*,*,#2920,.F.);
#4058=ORIENTED_EDGE('',*,*,#2923,.T.);
#4059=ORIENTED_EDGE('',*,*,#2926,.T.);
#4060=ORIENTED_EDGE('',*,*,#2882,.T.);
#4061=ORIENTED_EDGE('',*,*,#2872,.F.);
#4062=ORIENTED_EDGE('',*,*,#2876,.T.);
#4063=ORIENTED_EDGE('',*,*,#2879,.T.);
#4064=ORIENTED_EDGE('',*,*,#2887,.T.);
#4065=ORIENTED_EDGE('',*,*,#2904,.F.);
#4066=ORIENTED_EDGE('',*,*,#2907,.T.);
#4067=ORIENTED_EDGE('',*,*,#2910,.T.);
#4068=ORIENTED_EDGE('',*,*,#2898,.T.);
#4069=ORIENTED_EDGE('',*,*,#2888,.F.);
#4070=ORIENTED_EDGE('',*,*,#2892,.T.);
#4071=ORIENTED_EDGE('',*,*,#2895,.T.);
#4072=ORIENTED_EDGE('',*,*,#2903,.T.);
#4073=ORIENTED_EDGE('',*,*,#2928,.F.);
#4074=ORIENTED_EDGE('',*,*,#2931,.T.);
#4075=ORIENTED_EDGE('',*,*,#2934,.T.);
#4076=ORIENTED_EDGE('',*,*,#2939,.T.);
#4077=ORIENTED_EDGE('',*,*,#3024,.F.);
#4078=ORIENTED_EDGE('',*,*,#3027,.T.);
#4079=ORIENTED_EDGE('',*,*,#3030,.T.);
#4080=ORIENTED_EDGE('',*,*,#3035,.T.);
#4081=ORIENTED_EDGE('',*,*,#3052,.F.);
#4082=ORIENTED_EDGE('',*,*,#3055,.T.);
#4083=ORIENTED_EDGE('',*,*,#3058,.T.);
#4084=ORIENTED_EDGE('',*,*,#2637,.T.);
#4085=ORIENTED_EDGE('',*,*,#2644,.T.);
#4086=ORIENTED_EDGE('',*,*,#2641,.T.);
#4087=ORIENTED_EDGE('',*,*,#2628,.T.);
#4088=ORIENTED_EDGE('',*,*,#2652,.T.);
#4089=ORIENTED_EDGE('',*,*,#3060,.T.);
#4090=ORIENTED_EDGE('',*,*,#2653,.T.);
#4091=ORIENTED_EDGE('',*,*,#2646,.T.);
#4092=ORIENTED_EDGE('',*,*,#2624,.T.);
#4093=ORIENTED_EDGE('',*,*,#2640,.T.);
#4094=ORIENTED_EDGE('',*,*,#2660,.T.);
#4095=ORIENTED_EDGE('',*,*,#2632,.T.);
#4096=ORIENTED_EDGE('',*,*,#2753,.T.);
#4097=ORIENTED_EDGE('',*,*,#2760,.T.);
#4098=ORIENTED_EDGE('',*,*,#2757,.T.);
#4099=ORIENTED_EDGE('',*,*,#2744,.T.);
#4100=ORIENTED_EDGE('',*,*,#2768,.T.);
#4101=ORIENTED_EDGE('',*,*,#2812,.T.);
#4102=ORIENTED_EDGE('',*,*,#2769,.T.);
#4103=ORIENTED_EDGE('',*,*,#2762,.T.);
#4104=ORIENTED_EDGE('',*,*,#2785,.T.);
#4105=ORIENTED_EDGE('',*,*,#2840,.T.);
#4106=ORIENTED_EDGE('',*,*,#2789,.T.);
#4107=ORIENTED_EDGE('',*,*,#2776,.T.);
#4108=ORIENTED_EDGE('',*,*,#2805,.T.);
#4109=ORIENTED_EDGE('',*,*,#2824,.T.);
#4110=ORIENTED_EDGE('',*,*,#2809,.T.);
#4111=ORIENTED_EDGE('',*,*,#2796,.T.);
#4112=ORIENTED_EDGE('',*,*,#2820,.T.);
#4113=ORIENTED_EDGE('',*,*,#2828,.T.);
#4114=ORIENTED_EDGE('',*,*,#2821,.T.);
#4115=ORIENTED_EDGE('',*,*,#2814,.T.);
#4116=ORIENTED_EDGE('',*,*,#2772,.T.);
#4117=ORIENTED_EDGE('',*,*,#2788,.T.);
#4118=ORIENTED_EDGE('',*,*,#2826,.T.);
#4119=ORIENTED_EDGE('',*,*,#2780,.T.);
#4120=ORIENTED_EDGE('',*,*,#2836,.T.);
#4121=ORIENTED_EDGE('',*,*,#2940,.T.);
#4122=ORIENTED_EDGE('',*,*,#2837,.T.);
#4123=ORIENTED_EDGE('',*,*,#2830,.T.);
#4124=ORIENTED_EDGE('',*,*,#2740,.T.);
#4125=ORIENTED_EDGE('',*,*,#2756,.T.);
#4126=ORIENTED_EDGE('',*,*,#2842,.T.);
#4127=ORIENTED_EDGE('',*,*,#2748,.T.);
#4128=ORIENTED_EDGE('',*,*,#2948,.T.);
#4129=ORIENTED_EDGE('',*,*,#2964,.T.);
#4130=ORIENTED_EDGE('',*,*,#2949,.T.);
#4131=ORIENTED_EDGE('',*,*,#2942,.T.);
#4132=ORIENTED_EDGE('',*,*,#2656,.T.);
#4133=ORIENTED_EDGE('',*,*,#2667,.T.);
#4134=ORIENTED_EDGE('',*,*,#2956,.T.);
#4135=ORIENTED_EDGE('',*,*,#2662,.T.);
#4136=ORIENTED_EDGE('',*,*,#2952,.T.);
#4137=ORIENTED_EDGE('',*,*,#2963,.T.);
#4138=ORIENTED_EDGE('',*,*,#2966,.T.);
#4139=ORIENTED_EDGE('',*,*,#2958,.T.);
#4140=ORIENTED_EDGE('',*,*,#3064,.T.);
#4141=ORIENTED_EDGE('',*,*,#2792,.T.);
#4142=ORIENTED_EDGE('',*,*,#2808,.T.);
#4143=ORIENTED_EDGE('',*,*,#3062,.T.);
#4144=ORIENTED_EDGE('',*,*,#2800,.T.);
#4145=ORIENTED_EDGE('',*,*,#3033,.T.);
#4146=ORIENTED_EDGE('',*,*,#3031,.T.);
#4147=ORIENTED_EDGE('',*,*,#3028,.T.);
#4148=ORIENTED_EDGE('',*,*,#3025,.T.);
#4149=ORIENTED_EDGE('',*,*,#2937,.T.);
#4150=ORIENTED_EDGE('',*,*,#2935,.T.);
#4151=ORIENTED_EDGE('',*,*,#2932,.T.);
#4152=ORIENTED_EDGE('',*,*,#2929,.T.);
#4153=ORIENTED_EDGE('',*,*,#2901,.T.);
#4154=ORIENTED_EDGE('',*,*,#2896,.T.);
#4155=ORIENTED_EDGE('',*,*,#2893,.T.);
#4156=ORIENTED_EDGE('',*,*,#2890,.T.);
#4157=ORIENTED_EDGE('',*,*,#2900,.T.);
#4158=ORIENTED_EDGE('',*,*,#2911,.T.);
#4159=ORIENTED_EDGE('',*,*,#2908,.T.);
#4160=ORIENTED_EDGE('',*,*,#2905,.T.);
#4161=ORIENTED_EDGE('',*,*,#2885,.T.);
#4162=ORIENTED_EDGE('',*,*,#2880,.T.);
#4163=ORIENTED_EDGE('',*,*,#2877,.T.);
#4164=ORIENTED_EDGE('',*,*,#2874,.T.);
#4165=ORIENTED_EDGE('',*,*,#2884,.T.);
#4166=ORIENTED_EDGE('',*,*,#2927,.T.);
#4167=ORIENTED_EDGE('',*,*,#2924,.T.);
#4168=ORIENTED_EDGE('',*,*,#2921,.T.);
#4169=ORIENTED_EDGE('',*,*,#2869,.T.);
#4170=ORIENTED_EDGE('',*,*,#2867,.T.);
#4171=ORIENTED_EDGE('',*,*,#2864,.T.);
#4172=ORIENTED_EDGE('',*,*,#2861,.T.);
#4173=ORIENTED_EDGE('',*,*,#2857,.T.);
#4174=ORIENTED_EDGE('',*,*,#2852,.T.);
#4175=ORIENTED_EDGE('',*,*,#2849,.T.);
#4176=ORIENTED_EDGE('',*,*,#2846,.T.);
#4177=ORIENTED_EDGE('',*,*,#2856,.T.);
#4178=ORIENTED_EDGE('',*,*,#2919,.T.);
#4179=ORIENTED_EDGE('',*,*,#2916,.T.);
#4180=ORIENTED_EDGE('',*,*,#2913,.T.);
#4181=ORIENTED_EDGE('',*,*,#2581,.T.);
#4182=ORIENTED_EDGE('',*,*,#2576,.T.);
#4183=ORIENTED_EDGE('',*,*,#2573,.T.);
#4184=ORIENTED_EDGE('',*,*,#2570,.T.);
#4185=ORIENTED_EDGE('',*,*,#2580,.T.);
#4186=ORIENTED_EDGE('',*,*,#2623,.T.);
#4187=ORIENTED_EDGE('',*,*,#2620,.T.);
#4188=ORIENTED_EDGE('',*,*,#2617,.T.);
#4189=ORIENTED_EDGE('',*,*,#2601,.T.);
#4190=ORIENTED_EDGE('',*,*,#2599,.T.);
#4191=ORIENTED_EDGE('',*,*,#2596,.T.);
#4192=ORIENTED_EDGE('',*,*,#2593,.T.);
#4193=ORIENTED_EDGE('',*,*,#2553,.T.);
#4194=ORIENTED_EDGE('',*,*,#2548,.T.);
#4195=ORIENTED_EDGE('',*,*,#2545,.T.);
#4196=ORIENTED_EDGE('',*,*,#2542,.T.);
#4197=ORIENTED_EDGE('',*,*,#2552,.T.);
#4198=ORIENTED_EDGE('',*,*,#2591,.T.);
#4199=ORIENTED_EDGE('',*,*,#2588,.T.);
#4200=ORIENTED_EDGE('',*,*,#2585,.T.);
#4201=ORIENTED_EDGE('',*,*,#2565,.T.);
#4202=ORIENTED_EDGE('',*,*,#2563,.T.);
#4203=ORIENTED_EDGE('',*,*,#2560,.T.);
#4204=ORIENTED_EDGE('',*,*,#2557,.T.);
#4205=ORIENTED_EDGE('',*,*,#2537,.T.);
#4206=ORIENTED_EDGE('',*,*,#2532,.T.);
#4207=ORIENTED_EDGE('',*,*,#2529,.T.);
#4208=ORIENTED_EDGE('',*,*,#2526,.T.);
#4209=ORIENTED_EDGE('',*,*,#2536,.T.);
#4210=ORIENTED_EDGE('',*,*,#2612,.T.);
#4211=ORIENTED_EDGE('',*,*,#2609,.T.);
#4212=ORIENTED_EDGE('',*,*,#2606,.T.);
#4213=ORIENTED_EDGE('',*,*,#2615,.T.);
#4214=ORIENTED_EDGE('',*,*,#2739,.T.);
#4215=ORIENTED_EDGE('',*,*,#2736,.T.);
#4216=ORIENTED_EDGE('',*,*,#2733,.T.);
#4217=ORIENTED_EDGE('',*,*,#2729,.T.);
#4218=ORIENTED_EDGE('',*,*,#2727,.T.);
#4219=ORIENTED_EDGE('',*,*,#2724,.T.);
#4220=ORIENTED_EDGE('',*,*,#2721,.T.);
#4221=ORIENTED_EDGE('',*,*,#2681,.T.);
#4222=ORIENTED_EDGE('',*,*,#2676,.T.);
#4223=ORIENTED_EDGE('',*,*,#2673,.T.);
#4224=ORIENTED_EDGE('',*,*,#2670,.T.);
#4225=ORIENTED_EDGE('',*,*,#2680,.T.);
#4226=ORIENTED_EDGE('',*,*,#2719,.T.);
#4227=ORIENTED_EDGE('',*,*,#2716,.T.);
#4228=ORIENTED_EDGE('',*,*,#2713,.T.);
#4229=ORIENTED_EDGE('',*,*,#2709,.T.);
#4230=ORIENTED_EDGE('',*,*,#2707,.T.);
#4231=ORIENTED_EDGE('',*,*,#2704,.T.);
#4232=ORIENTED_EDGE('',*,*,#2701,.T.);
#4233=ORIENTED_EDGE('',*,*,#2697,.T.);
#4234=ORIENTED_EDGE('',*,*,#2692,.T.);
#4235=ORIENTED_EDGE('',*,*,#2689,.T.);
#4236=ORIENTED_EDGE('',*,*,#2686,.T.);
#4237=ORIENTED_EDGE('',*,*,#2696,.T.);
#4238=ORIENTED_EDGE('',*,*,#3043,.T.);
#4239=ORIENTED_EDGE('',*,*,#3040,.T.);
#4240=ORIENTED_EDGE('',*,*,#3037,.T.);
#4241=ORIENTED_EDGE('',*,*,#3009,.T.);
#4242=ORIENTED_EDGE('',*,*,#3004,.T.);
#4243=ORIENTED_EDGE('',*,*,#3001,.T.);
#4244=ORIENTED_EDGE('',*,*,#2998,.T.);
#4245=ORIENTED_EDGE('',*,*,#3008,.T.);
#4246=ORIENTED_EDGE('',*,*,#3051,.T.);
#4247=ORIENTED_EDGE('',*,*,#3048,.T.);
#4248=ORIENTED_EDGE('',*,*,#3045,.T.);
#4249=ORIENTED_EDGE('',*,*,#3021,.T.);
#4250=ORIENTED_EDGE('',*,*,#3019,.T.);
#4251=ORIENTED_EDGE('',*,*,#3016,.T.);
#4252=ORIENTED_EDGE('',*,*,#3013,.T.);
#4253=ORIENTED_EDGE('',*,*,#2993,.T.);
#4254=ORIENTED_EDGE('',*,*,#2991,.T.);
#4255=ORIENTED_EDGE('',*,*,#2988,.T.);
#4256=ORIENTED_EDGE('',*,*,#2985,.T.);
#4257=ORIENTED_EDGE('',*,*,#2981,.T.);
#4258=ORIENTED_EDGE('',*,*,#2976,.T.);
#4259=ORIENTED_EDGE('',*,*,#2973,.T.);
#4260=ORIENTED_EDGE('',*,*,#2970,.T.);
#4261=ORIENTED_EDGE('',*,*,#2980,.T.);
#4262=ORIENTED_EDGE('',*,*,#3059,.T.);
#4263=ORIENTED_EDGE('',*,*,#3056,.T.);
#4264=ORIENTED_EDGE('',*,*,#3053,.T.);
#4265=ORIENTED_EDGE('',*,*,#2634,.T.);
#4266=ORIENTED_EDGE('',*,*,#2661,.T.);
#4267=ORIENTED_EDGE('',*,*,#2638,.T.);
#4268=ORIENTED_EDGE('',*,*,#2626,.T.);
#4269=ORIENTED_EDGE('',*,*,#2630,.T.);
#4270=ORIENTED_EDGE('',*,*,#2643,.T.);
#4271=ORIENTED_EDGE('',*,*,#2645,.T.);
#4272=ORIENTED_EDGE('',*,*,#2635,.T.);
#4273=ORIENTED_EDGE('',*,*,#2664,.T.);
#4274=ORIENTED_EDGE('',*,*,#2957,.T.);
#4275=ORIENTED_EDGE('',*,*,#2665,.T.);
#4276=ORIENTED_EDGE('',*,*,#2658,.T.);
#4277=ORIENTED_EDGE('',*,*,#2750,.T.);
#4278=ORIENTED_EDGE('',*,*,#2843,.T.);
#4279=ORIENTED_EDGE('',*,*,#2754,.T.);
#4280=ORIENTED_EDGE('',*,*,#2742,.T.);
#4281=ORIENTED_EDGE('',*,*,#2746,.T.);
#4282=ORIENTED_EDGE('',*,*,#2759,.T.);
#4283=ORIENTED_EDGE('',*,*,#2761,.T.);
#4284=ORIENTED_EDGE('',*,*,#2751,.T.);
#4285=ORIENTED_EDGE('',*,*,#2782,.T.);
#4286=ORIENTED_EDGE('',*,*,#2827,.T.);
#4287=ORIENTED_EDGE('',*,*,#2786,.T.);
#4288=ORIENTED_EDGE('',*,*,#2774,.T.);
#4289=ORIENTED_EDGE('',*,*,#2802,.T.);
#4290=ORIENTED_EDGE('',*,*,#3063,.T.);
#4291=ORIENTED_EDGE('',*,*,#2806,.T.);
#4292=ORIENTED_EDGE('',*,*,#2794,.T.);
#4293=ORIENTED_EDGE('',*,*,#2764,.T.);
#4294=ORIENTED_EDGE('',*,*,#2771,.T.);
#4295=ORIENTED_EDGE('',*,*,#2813,.T.);
#4296=ORIENTED_EDGE('',*,*,#2766,.T.);
#4297=ORIENTED_EDGE('',*,*,#2798,.T.);
#4298=ORIENTED_EDGE('',*,*,#2811,.T.);
#4299=ORIENTED_EDGE('',*,*,#2825,.T.);
#4300=ORIENTED_EDGE('',*,*,#2803,.T.);
#4301=ORIENTED_EDGE('',*,*,#2816,.T.);
#4302=ORIENTED_EDGE('',*,*,#2823,.T.);
#4303=ORIENTED_EDGE('',*,*,#2829,.T.);
#4304=ORIENTED_EDGE('',*,*,#2818,.T.);
#4305=ORIENTED_EDGE('',*,*,#2778,.T.);
#4306=ORIENTED_EDGE('',*,*,#2791,.T.);
#4307=ORIENTED_EDGE('',*,*,#2841,.T.);
#4308=ORIENTED_EDGE('',*,*,#2783,.T.);
#4309=ORIENTED_EDGE('',*,*,#2832,.T.);
#4310=ORIENTED_EDGE('',*,*,#2839,.T.);
#4311=ORIENTED_EDGE('',*,*,#2941,.T.);
#4312=ORIENTED_EDGE('',*,*,#2834,.T.);
#4313=ORIENTED_EDGE('',*,*,#2960,.T.);
#4314=ORIENTED_EDGE('',*,*,#2967,.T.);
#4315=ORIENTED_EDGE('',*,*,#2961,.T.);
#4316=ORIENTED_EDGE('',*,*,#2954,.T.);
#4317=ORIENTED_EDGE('',*,*,#2944,.T.);
#4318=ORIENTED_EDGE('',*,*,#2951,.T.);
#4319=ORIENTED_EDGE('',*,*,#2965,.T.);
#4320=ORIENTED_EDGE('',*,*,#2946,.T.);
#4321=ORIENTED_EDGE('',*,*,#3066,.T.);
#4322=ORIENTED_EDGE('',*,*,#2648,.T.);
#4323=ORIENTED_EDGE('',*,*,#2655,.T.);
#4324=ORIENTED_EDGE('',*,*,#3061,.T.);
#4325=ORIENTED_EDGE('',*,*,#2650,.T.);
#4672=PLANE('',#5204);
#4673=PLANE('',#5205);
#4674=PLANE('',#5206);
#4675=PLANE('',#5213);
#4676=PLANE('',#5214);
#4677=PLANE('',#5215);
#4678=PLANE('',#5222);
#4679=PLANE('',#5223);
#4680=PLANE('',#5224);
#4681=PLANE('',#5228);
#4682=PLANE('',#5229);
#4683=PLANE('',#5230);
#4684=PLANE('',#5237);
#4685=PLANE('',#5238);
#4686=PLANE('',#5239);
#4687=PLANE('',#5240);
#4688=PLANE('',#5241);
#4689=PLANE('',#5242);
#4690=PLANE('',#5246);
#4691=PLANE('',#5247);
#4692=PLANE('',#5248);
#4693=PLANE('',#5252);
#4694=PLANE('',#5253);
#4695=PLANE('',#5254);
#4696=PLANE('',#5255);
#4697=PLANE('',#5256);
#4698=PLANE('',#5269);
#4699=PLANE('',#5270);
#4700=PLANE('',#5277);
#4701=PLANE('',#5278);
#4702=PLANE('',#5285);
#4703=PLANE('',#5286);
#4704=PLANE('',#5287);
#4705=PLANE('',#5294);
#4706=PLANE('',#5295);
#4707=PLANE('',#5296);
#4708=PLANE('',#5303);
#4709=PLANE('',#5304);
#4710=PLANE('',#5305);
#4711=PLANE('',#5309);
#4712=PLANE('',#5310);
#4713=PLANE('',#5311);
#4714=PLANE('',#5312);
#4715=PLANE('',#5313);
#4716=PLANE('',#5314);
#4717=PLANE('',#5318);
#4718=PLANE('',#5319);
#4719=PLANE('',#5320);
#4720=PLANE('',#5321);
#4721=PLANE('',#5322);
#4722=PLANE('',#5335);
#4723=PLANE('',#5336);
#4724=PLANE('',#5343);
#4725=PLANE('',#5344);
#4726=PLANE('',#5357);
#4727=PLANE('',#5358);
#4728=PLANE('',#5371);
#4729=PLANE('',#5372);
#4730=PLANE('',#5379);
#4731=PLANE('',#5380);
#4732=PLANE('',#5381);
#4733=PLANE('',#5382);
#4734=PLANE('',#5389);
#4735=PLANE('',#5390);
#4736=PLANE('',#5391);
#4737=PLANE('',#5392);
#4738=PLANE('',#5393);
#4739=PLANE('',#5400);
#4740=PLANE('',#5401);
#4741=PLANE('',#5402);
#4742=PLANE('',#5406);
#4743=PLANE('',#5407);
#4744=PLANE('',#5408);
#4745=PLANE('',#5415);
#4746=PLANE('',#5416);
#4747=PLANE('',#5417);
#4748=PLANE('',#5424);
#4749=PLANE('',#5425);
#4750=PLANE('',#5426);
#4751=PLANE('',#5427);
#4752=PLANE('',#5428);
#4753=PLANE('',#5429);
#4754=PLANE('',#5430);
#4755=PLANE('',#5431);
#4756=PLANE('',#5432);
#4757=PLANE('',#5433);
#4758=PLANE('',#5434);
#4759=PLANE('',#5435);
#4760=PLANE('',#5439);
#4761=PLANE('',#5440);
#4762=PLANE('',#5447);
#4763=PLANE('',#5448);
#4764=PLANE('',#5455);
#4765=PLANE('',#5456);
#4766=PLANE('',#5457);
#4767=PLANE('',#5458);
#4768=PLANE('',#5459);
#4769=PLANE('',#5466);
#4770=PLANE('',#5467);
#4771=PLANE('',#5468);
#4772=PLANE('',#5472);
#4773=PLANE('',#5473);
#4774=PLANE('',#5474);
#4775=PLANE('',#5481);
#4776=PLANE('',#5482);
#4777=PLANE('',#5483);
#4778=PLANE('',#5487);
#4779=PLANE('',#5488);
#4780=PLANE('',#5489);
#4781=PLANE('',#5493);
#4782=PLANE('',#5494);
#4783=PLANE('',#5495);
#4784=PLANE('',#5496);
#4785=PLANE('',#5497);
#4786=PLANE('',#5498);
#4787=PLANE('',#5499);
#4788=PLANE('',#5500);
#4789=PLANE('',#5501);
#4790=PLANE('',#5502);
#4791=PLANE('',#5503);
#4792=PLANE('',#5507);
#4793=PLANE('',#5508);
#4837=ADVANCED_FACE('',(#475),#4672,.T.);
#4838=ADVANCED_FACE('',(#476),#4673,.T.);
#4839=ADVANCED_FACE('',(#477),#4674,.T.);
#4840=ADVANCED_FACE('',(#478),#396,.T.);
#4841=ADVANCED_FACE('',(#479),#397,.T.);
#4842=ADVANCED_FACE('',(#480),#4675,.T.);
#4843=ADVANCED_FACE('',(#481),#4676,.T.);
#4844=ADVANCED_FACE('',(#482),#4677,.T.);
#4845=ADVANCED_FACE('',(#483),#398,.T.);
#4846=ADVANCED_FACE('',(#484),#399,.T.);
#4847=ADVANCED_FACE('',(#485),#4678,.T.);
#4848=ADVANCED_FACE('',(#486),#4679,.T.);
#4849=ADVANCED_FACE('',(#487),#4680,.T.);
#4850=ADVANCED_FACE('',(#488),#400,.T.);
#4851=ADVANCED_FACE('',(#489),#4681,.T.);
#4852=ADVANCED_FACE('',(#490),#4682,.T.);
#4853=ADVANCED_FACE('',(#491),#4683,.T.);
#4854=ADVANCED_FACE('',(#492),#401,.T.);
#4855=ADVANCED_FACE('',(#493),#402,.T.);
#4856=ADVANCED_FACE('',(#494),#4684,.T.);
#4857=ADVANCED_FACE('',(#495),#4685,.T.);
#4858=ADVANCED_FACE('',(#496),#4686,.T.);
#4859=ADVANCED_FACE('',(#497),#4687,.T.);
#4860=ADVANCED_FACE('',(#498),#4688,.T.);
#4861=ADVANCED_FACE('',(#499),#4689,.T.);
#4862=ADVANCED_FACE('',(#500),#403,.T.);
#4863=ADVANCED_FACE('',(#501),#4690,.T.);
#4864=ADVANCED_FACE('',(#502),#4691,.T.);
#4865=ADVANCED_FACE('',(#503),#4692,.T.);
#4866=ADVANCED_FACE('',(#504),#404,.T.);
#4867=ADVANCED_FACE('',(#505),#4693,.T.);
#4868=ADVANCED_FACE('',(#506),#4694,.T.);
#4869=ADVANCED_FACE('',(#507),#4695,.T.);
#4870=ADVANCED_FACE('',(#508),#4696,.T.);
#4871=ADVANCED_FACE('',(#509),#4697,.T.);
#4872=ADVANCED_FACE('',(#510),#405,.F.);
#4873=ADVANCED_FACE('',(#511),#406,.F.);
#4874=ADVANCED_FACE('',(#512),#407,.T.);
#4875=ADVANCED_FACE('',(#513),#408,.T.);
#4876=ADVANCED_FACE('',(#514),#4698,.T.);
#4877=ADVANCED_FACE('',(#515),#4699,.T.);
#4878=ADVANCED_FACE('',(#516),#409,.F.);
#4879=ADVANCED_FACE('',(#517),#410,.T.);
#4880=ADVANCED_FACE('',(#518),#4700,.T.);
#4881=ADVANCED_FACE('',(#519),#4701,.T.);
#4882=ADVANCED_FACE('',(#520),#411,.F.);
#4883=ADVANCED_FACE('',(#521),#412,.T.);
#4884=ADVANCED_FACE('',(#522),#4702,.T.);
#4885=ADVANCED_FACE('',(#523),#4703,.T.);
#4886=ADVANCED_FACE('',(#524),#4704,.T.);
#4887=ADVANCED_FACE('',(#525),#413,.T.);
#4888=ADVANCED_FACE('',(#526),#414,.T.);
#4889=ADVANCED_FACE('',(#527),#4705,.T.);
#4890=ADVANCED_FACE('',(#528),#4706,.T.);
#4891=ADVANCED_FACE('',(#529),#4707,.T.);
#4892=ADVANCED_FACE('',(#530),#415,.T.);
#4893=ADVANCED_FACE('',(#531),#416,.T.);
#4894=ADVANCED_FACE('',(#532),#4708,.T.);
#4895=ADVANCED_FACE('',(#533),#4709,.T.);
#4896=ADVANCED_FACE('',(#534),#4710,.T.);
#4897=ADVANCED_FACE('',(#535),#417,.T.);
#4898=ADVANCED_FACE('',(#536),#4711,.T.);
#4899=ADVANCED_FACE('',(#537),#4712,.T.);
#4900=ADVANCED_FACE('',(#538),#4713,.T.);
#4901=ADVANCED_FACE('',(#539),#4714,.T.);
#4902=ADVANCED_FACE('',(#540),#4715,.T.);
#4903=ADVANCED_FACE('',(#541),#4716,.T.);
#4904=ADVANCED_FACE('',(#542),#418,.T.);
#4905=ADVANCED_FACE('',(#543),#4717,.T.);
#4906=ADVANCED_FACE('',(#544),#4718,.T.);
#4907=ADVANCED_FACE('',(#545),#4719,.T.);
#4908=ADVANCED_FACE('',(#546),#4720,.T.);
#4909=ADVANCED_FACE('',(#547),#4721,.T.);
#4910=ADVANCED_FACE('',(#548),#419,.F.);
#4911=ADVANCED_FACE('',(#549),#420,.F.);
#4912=ADVANCED_FACE('',(#550),#421,.T.);
#4913=ADVANCED_FACE('',(#551),#422,.T.);
#4914=ADVANCED_FACE('',(#552),#4722,.T.);
#4915=ADVANCED_FACE('',(#553),#4723,.T.);
#4916=ADVANCED_FACE('',(#554),#423,.F.);
#4917=ADVANCED_FACE('',(#555),#424,.T.);
#4918=ADVANCED_FACE('',(#556),#4724,.T.);
#4919=ADVANCED_FACE('',(#557),#4725,.T.);
#4920=ADVANCED_FACE('',(#558),#425,.F.);
#4921=ADVANCED_FACE('',(#559),#426,.F.);
#4922=ADVANCED_FACE('',(#560),#427,.T.);
#4923=ADVANCED_FACE('',(#561),#428,.T.);
#4924=ADVANCED_FACE('',(#562),#4726,.T.);
#4925=ADVANCED_FACE('',(#563),#4727,.T.);
#4926=ADVANCED_FACE('',(#564),#429,.F.);
#4927=ADVANCED_FACE('',(#565),#430,.F.);
#4928=ADVANCED_FACE('',(#566),#431,.T.);
#4929=ADVANCED_FACE('',(#567),#432,.T.);
#4930=ADVANCED_FACE('',(#568),#4728,.T.);
#4931=ADVANCED_FACE('',(#569),#4729,.T.);
#4932=ADVANCED_FACE('',(#570),#433,.F.);
#4933=ADVANCED_FACE('',(#571),#434,.T.);
#4934=ADVANCED_FACE('',(#572),#4730,.T.);
#4935=ADVANCED_FACE('',(#573),#4731,.T.);
#4936=ADVANCED_FACE('',(#574),#4732,.T.);
#4937=ADVANCED_FACE('',(#575),#4733,.T.);
#4938=ADVANCED_FACE('',(#576),#435,.F.);
#4939=ADVANCED_FACE('',(#577),#436,.T.);
#4940=ADVANCED_FACE('',(#578),#4734,.T.);
#4941=ADVANCED_FACE('',(#579),#4735,.T.);
#4942=ADVANCED_FACE('',(#580),#4736,.T.);
#4943=ADVANCED_FACE('',(#581),#4737,.T.);
#4944=ADVANCED_FACE('',(#582),#4738,.T.);
#4945=ADVANCED_FACE('',(#583),#437,.T.);
#4946=ADVANCED_FACE('',(#584),#438,.T.);
#4947=ADVANCED_FACE('',(#585),#4739,.T.);
#4948=ADVANCED_FACE('',(#586),#4740,.T.);
#4949=ADVANCED_FACE('',(#587),#4741,.T.);
#4950=ADVANCED_FACE('',(#588),#439,.T.);
#4951=ADVANCED_FACE('',(#589),#4742,.T.);
#4952=ADVANCED_FACE('',(#590),#4743,.T.);
#4953=ADVANCED_FACE('',(#591),#4744,.T.);
#4954=ADVANCED_FACE('',(#592),#440,.T.);
#4955=ADVANCED_FACE('',(#593),#441,.T.);
#4956=ADVANCED_FACE('',(#594),#4745,.T.);
#4957=ADVANCED_FACE('',(#595),#4746,.T.);
#4958=ADVANCED_FACE('',(#596),#4747,.T.);
#4959=ADVANCED_FACE('',(#597),#442,.T.);
#4960=ADVANCED_FACE('',(#598),#443,.T.);
#4961=ADVANCED_FACE('',(#599),#4748,.T.);
#4962=ADVANCED_FACE('',(#600),#4749,.T.);
#4963=ADVANCED_FACE('',(#601),#4750,.T.);
#4964=ADVANCED_FACE('',(#602),#4751,.T.);
#4965=ADVANCED_FACE('',(#603),#4752,.T.);
#4966=ADVANCED_FACE('',(#604),#4753,.T.);
#4967=ADVANCED_FACE('',(#605),#4754,.T.);
#4968=ADVANCED_FACE('',(#606),#4755,.T.);
#4969=ADVANCED_FACE('',(#607),#4756,.T.);
#4970=ADVANCED_FACE('',(#608),#4757,.T.);
#4971=ADVANCED_FACE('',(#609),#4758,.T.);
#4972=ADVANCED_FACE('',(#610),#4759,.T.);
#4973=ADVANCED_FACE('',(#611),#444,.T.);
#4974=ADVANCED_FACE('',(#612),#4760,.T.);
#4975=ADVANCED_FACE('',(#613),#4761,.T.);
#4976=ADVANCED_FACE('',(#614),#445,.F.);
#4977=ADVANCED_FACE('',(#615),#446,.T.);
#4978=ADVANCED_FACE('',(#616),#4762,.T.);
#4979=ADVANCED_FACE('',(#617),#4763,.T.);
#4980=ADVANCED_FACE('',(#618),#447,.F.);
#4981=ADVANCED_FACE('',(#619),#448,.T.);
#4982=ADVANCED_FACE('',(#620),#4764,.T.);
#4983=ADVANCED_FACE('',(#621),#4765,.T.);
#4984=ADVANCED_FACE('',(#622),#4766,.T.);
#4985=ADVANCED_FACE('',(#623),#4767,.T.);
#4986=ADVANCED_FACE('',(#624),#4768,.T.);
#4987=ADVANCED_FACE('',(#625),#449,.T.);
#4988=ADVANCED_FACE('',(#626),#450,.T.);
#4989=ADVANCED_FACE('',(#627),#4769,.T.);
#4990=ADVANCED_FACE('',(#628),#4770,.T.);
#4991=ADVANCED_FACE('',(#629),#4771,.T.);
#4992=ADVANCED_FACE('',(#630),#451,.T.);
#4993=ADVANCED_FACE('',(#631),#4772,.T.);
#4994=ADVANCED_FACE('',(#632),#4773,.T.);
#4995=ADVANCED_FACE('',(#633),#4774,.T.);
#4996=ADVANCED_FACE('',(#634),#452,.T.);
#4997=ADVANCED_FACE('',(#635),#453,.T.);
#4998=ADVANCED_FACE('',(#636),#4775,.T.);
#4999=ADVANCED_FACE('',(#637),#4776,.T.);
#5000=ADVANCED_FACE('',(#638),#4777,.T.);
#5001=ADVANCED_FACE('',(#639),#454,.T.);
#5002=ADVANCED_FACE('',(#640),#4778,.T.);
#5003=ADVANCED_FACE('',(#641),#4779,.T.);
#5004=ADVANCED_FACE('',(#642),#4780,.T.);
#5005=ADVANCED_FACE('',(#643),#455,.T.);
#5006=ADVANCED_FACE('',(#644),#4781,.T.);
#5007=ADVANCED_FACE('',(#645),#4782,.T.);
#5008=ADVANCED_FACE('',(#646),#4783,.T.);
#5009=ADVANCED_FACE('',(#647),#4784,.T.);
#5010=ADVANCED_FACE('',(#648),#4785,.T.);
#5011=ADVANCED_FACE('',(#649),#4786,.T.);
#5012=ADVANCED_FACE('',(#650),#4787,.T.);
#5013=ADVANCED_FACE('',(#651),#4788,.T.);
#5014=ADVANCED_FACE('',(#652),#4789,.T.);
#5015=ADVANCED_FACE('',(#653),#4790,.T.);
#5016=ADVANCED_FACE('',(#654),#4791,.T.);
#5017=ADVANCED_FACE('',(#655),#456,.F.);
#5018=ADVANCED_FACE('',(#656,#114,#115,#116,#117,#118,#119,#120,#121,#122,
#123,#124,#125,#126,#127,#128,#129),#4792,.T.);
#5019=ADVANCED_FACE('',(#657,#130,#131,#132,#133,#134,#135,#136,#137,#138,
#139,#140,#141,#142,#143,#144,#145),#4793,.F.);
#5114=CLOSED_SHELL('',(#4837,#4838,#4839,#4840,#4841,#4842,#4843,#4844,
#4845,#4846,#4847,#4848,#4849,#4850,#4851,#4852,#4853,#4854,#4855,#4856,
#4857,#4858,#4859,#4860,#4861,#4862,#4863,#4864,#4865,#4866,#4867,#4868,
#4869,#4870,#4871,#4872,#4873,#4874,#4875,#4876,#4877,#4878,#4879,#4880,
#4881,#4882,#4883,#4884,#4885,#4886,#4887,#4888,#4889,#4890,#4891,#4892,
#4893,#4894,#4895,#4896,#4897,#4898,#4899,#4900,#4901,#4902,#4903,#4904,
#4905,#4906,#4907,#4908,#4909,#4910,#4911,#4912,#4913,#4914,#4915,#4916,
#4917,#4918,#4919,#4920,#4921,#4922,#4923,#4924,#4925,#4926,#4927,#4928,
#4929,#4930,#4931,#4932,#4933,#4934,#4935,#4936,#4937,#4938,#4939,#4940,
#4941,#4942,#4943,#4944,#4945,#4946,#4947,#4948,#4949,#4950,#4951,#4952,
#4953,#4954,#4955,#4956,#4957,#4958,#4959,#4960,#4961,#4962,#4963,#4964,
#4965,#4966,#4967,#4968,#4969,#4970,#4971,#4972,#4973,#4974,#4975,#4976,
#4977,#4978,#4979,#4980,#4981,#4982,#4983,#4984,#4985,#4986,#4987,#4988,
#4989,#4990,#4991,#4992,#4993,#4994,#4995,#4996,#4997,#4998,#4999,#5000,
#5001,#5002,#5003,#5004,#5005,#5006,#5007,#5008,#5009,#5010,#5011,#5012,
#5013,#5014,#5015,#5016,#5017,#5018,#5019));
#5203=AXIS2_PLACEMENT_3D('',#7248,#5724,#5725);
#5204=AXIS2_PLACEMENT_3D('',#7249,#5726,#5727);
#5205=AXIS2_PLACEMENT_3D('',#7258,#5732,#5733);
#5206=AXIS2_PLACEMENT_3D('',#7264,#5737,#5738);
#5207=AXIS2_PLACEMENT_3D('',#7270,#5742,#5743);
#5208=AXIS2_PLACEMENT_3D('',#7272,#5744,#5745);
#5209=AXIS2_PLACEMENT_3D('',#7275,#5747,#5748);
#5210=AXIS2_PLACEMENT_3D('',#7276,#5749,#5750);
#5211=AXIS2_PLACEMENT_3D('',#7278,#5751,#5752);
#5212=AXIS2_PLACEMENT_3D('',#7281,#5754,#5755);
#5213=AXIS2_PLACEMENT_3D('',#7282,#5756,#5757);
#5214=AXIS2_PLACEMENT_3D('',#7291,#5762,#5763);
#5215=AXIS2_PLACEMENT_3D('',#7297,#5767,#5768);
#5216=AXIS2_PLACEMENT_3D('',#7303,#5772,#5773);
#5217=AXIS2_PLACEMENT_3D('',#7305,#5774,#5775);
#5218=AXIS2_PLACEMENT_3D('',#7308,#5777,#5778);
#5219=AXIS2_PLACEMENT_3D('',#7309,#5779,#5780);
#5220=AXIS2_PLACEMENT_3D('',#7311,#5781,#5782);
#5221=AXIS2_PLACEMENT_3D('',#7314,#5784,#5785);
#5222=AXIS2_PLACEMENT_3D('',#7315,#5786,#5787);
#5223=AXIS2_PLACEMENT_3D('',#7321,#5791,#5792);
#5224=AXIS2_PLACEMENT_3D('',#7327,#5796,#5797);
#5225=AXIS2_PLACEMENT_3D('',#7333,#5801,#5802);
#5226=AXIS2_PLACEMENT_3D('',#7335,#5803,#5804);
#5227=AXIS2_PLACEMENT_3D('',#7338,#5806,#5807);
#5228=AXIS2_PLACEMENT_3D('',#7339,#5808,#5809);
#5229=AXIS2_PLACEMENT_3D('',#7348,#5814,#5815);
#5230=AXIS2_PLACEMENT_3D('',#7354,#5819,#5820);
#5231=AXIS2_PLACEMENT_3D('',#7360,#5824,#5825);
#5232=AXIS2_PLACEMENT_3D('',#7362,#5826,#5827);
#5233=AXIS2_PLACEMENT_3D('',#7365,#5829,#5830);
#5234=AXIS2_PLACEMENT_3D('',#7366,#5831,#5832);
#5235=AXIS2_PLACEMENT_3D('',#7368,#5833,#5834);
#5236=AXIS2_PLACEMENT_3D('',#7371,#5836,#5837);
#5237=AXIS2_PLACEMENT_3D('',#7372,#5838,#5839);
#5238=AXIS2_PLACEMENT_3D('',#7378,#5843,#5844);
#5239=AXIS2_PLACEMENT_3D('',#7384,#5848,#5849);
#5240=AXIS2_PLACEMENT_3D('',#7387,#5852,#5853);
#5241=AXIS2_PLACEMENT_3D('',#7393,#5857,#5858);
#5242=AXIS2_PLACEMENT_3D('',#7399,#5862,#5863);
#5243=AXIS2_PLACEMENT_3D('',#7405,#5867,#5868);
#5244=AXIS2_PLACEMENT_3D('',#7407,#5869,#5870);
#5245=AXIS2_PLACEMENT_3D('',#7410,#5872,#5873);
#5246=AXIS2_PLACEMENT_3D('',#7411,#5874,#5875);
#5247=AXIS2_PLACEMENT_3D('',#7420,#5880,#5881);
#5248=AXIS2_PLACEMENT_3D('',#7426,#5885,#5886);
#5249=AXIS2_PLACEMENT_3D('',#7429,#5889,#5890);
#5250=AXIS2_PLACEMENT_3D('',#7431,#5891,#5892);
#5251=AXIS2_PLACEMENT_3D('',#7434,#5894,#5895);
#5252=AXIS2_PLACEMENT_3D('',#7435,#5896,#5897);
#5253=AXIS2_PLACEMENT_3D('',#7441,#5901,#5902);
#5254=AXIS2_PLACEMENT_3D('',#7447,#5906,#5907);
#5255=AXIS2_PLACEMENT_3D('',#7450,#5910,#5911);
#5256=AXIS2_PLACEMENT_3D('',#7459,#5916,#5917);
#5257=AXIS2_PLACEMENT_3D('',#7468,#5922,#5923);
#5258=AXIS2_PLACEMENT_3D('',#7470,#5924,#5925);
#5259=AXIS2_PLACEMENT_3D('',#7473,#5927,#5928);
#5260=AXIS2_PLACEMENT_3D('',#7474,#5929,#5930);
#5261=AXIS2_PLACEMENT_3D('',#7476,#5931,#5932);
#5262=AXIS2_PLACEMENT_3D('',#7479,#5934,#5935);
#5263=AXIS2_PLACEMENT_3D('',#7480,#5936,#5937);
#5264=AXIS2_PLACEMENT_3D('',#7482,#5938,#5939);
#5265=AXIS2_PLACEMENT_3D('',#7485,#5941,#5942);
#5266=AXIS2_PLACEMENT_3D('',#7486,#5943,#5944);
#5267=AXIS2_PLACEMENT_3D('',#7488,#5945,#5946);
#5268=AXIS2_PLACEMENT_3D('',#7491,#5948,#5949);
#5269=AXIS2_PLACEMENT_3D('',#7492,#5950,#5951);
#5270=AXIS2_PLACEMENT_3D('',#7495,#5954,#5955);
#5271=AXIS2_PLACEMENT_3D('',#7504,#5960,#5961);
#5272=AXIS2_PLACEMENT_3D('',#7506,#5962,#5963);
#5273=AXIS2_PLACEMENT_3D('',#7509,#5965,#5966);
#5274=AXIS2_PLACEMENT_3D('',#7510,#5967,#5968);
#5275=AXIS2_PLACEMENT_3D('',#7512,#5969,#5970);
#5276=AXIS2_PLACEMENT_3D('',#7515,#5972,#5973);
#5277=AXIS2_PLACEMENT_3D('',#7516,#5974,#5975);
#5278=AXIS2_PLACEMENT_3D('',#7525,#5980,#5981);
#5279=AXIS2_PLACEMENT_3D('',#7528,#5984,#5985);
#5280=AXIS2_PLACEMENT_3D('',#7530,#5986,#5987);
#5281=AXIS2_PLACEMENT_3D('',#7533,#5989,#5990);
#5282=AXIS2_PLACEMENT_3D('',#7534,#5991,#5992);
#5283=AXIS2_PLACEMENT_3D('',#7536,#5993,#5994);
#5284=AXIS2_PLACEMENT_3D('',#7539,#5996,#5997);
#5285=AXIS2_PLACEMENT_3D('',#7540,#5998,#5999);
#5286=AXIS2_PLACEMENT_3D('',#7549,#6004,#6005);
#5287=AXIS2_PLACEMENT_3D('',#7555,#6009,#6010);
#5288=AXIS2_PLACEMENT_3D('',#7561,#6014,#6015);
#5289=AXIS2_PLACEMENT_3D('',#7563,#6016,#6017);
#5290=AXIS2_PLACEMENT_3D('',#7566,#6019,#6020);
#5291=AXIS2_PLACEMENT_3D('',#7567,#6021,#6022);
#5292=AXIS2_PLACEMENT_3D('',#7569,#6023,#6024);
#5293=AXIS2_PLACEMENT_3D('',#7572,#6026,#6027);
#5294=AXIS2_PLACEMENT_3D('',#7573,#6028,#6029);
#5295=AXIS2_PLACEMENT_3D('',#7582,#6034,#6035);
#5296=AXIS2_PLACEMENT_3D('',#7588,#6039,#6040);
#5297=AXIS2_PLACEMENT_3D('',#7594,#6044,#6045);
#5298=AXIS2_PLACEMENT_3D('',#7596,#6046,#6047);
#5299=AXIS2_PLACEMENT_3D('',#7599,#6049,#6050);
#5300=AXIS2_PLACEMENT_3D('',#7600,#6051,#6052);
#5301=AXIS2_PLACEMENT_3D('',#7602,#6053,#6054);
#5302=AXIS2_PLACEMENT_3D('',#7605,#6056,#6057);
#5303=AXIS2_PLACEMENT_3D('',#7606,#6058,#6059);
#5304=AXIS2_PLACEMENT_3D('',#7612,#6063,#6064);
#5305=AXIS2_PLACEMENT_3D('',#7618,#6068,#6069);
#5306=AXIS2_PLACEMENT_3D('',#7624,#6073,#6074);
#5307=AXIS2_PLACEMENT_3D('',#7626,#6075,#6076);
#5308=AXIS2_PLACEMENT_3D('',#7629,#6078,#6079);
#5309=AXIS2_PLACEMENT_3D('',#7630,#6080,#6081);
#5310=AXIS2_PLACEMENT_3D('',#7636,#6085,#6086);
#5311=AXIS2_PLACEMENT_3D('',#7642,#6090,#6091);
#5312=AXIS2_PLACEMENT_3D('',#7645,#6094,#6095);
#5313=AXIS2_PLACEMENT_3D('',#7651,#6099,#6100);
#5314=AXIS2_PLACEMENT_3D('',#7657,#6104,#6105);
#5315=AXIS2_PLACEMENT_3D('',#7663,#6109,#6110);
#5316=AXIS2_PLACEMENT_3D('',#7665,#6111,#6112);
#5317=AXIS2_PLACEMENT_3D('',#7668,#6114,#6115);
#5318=AXIS2_PLACEMENT_3D('',#7669,#6116,#6117);
#5319=AXIS2_PLACEMENT_3D('',#7675,#6121,#6122);
#5320=AXIS2_PLACEMENT_3D('',#7681,#6126,#6127);
#5321=AXIS2_PLACEMENT_3D('',#7684,#6130,#6131);
#5322=AXIS2_PLACEMENT_3D('',#7693,#6136,#6137);
#5323=AXIS2_PLACEMENT_3D('',#7702,#6142,#6143);
#5324=AXIS2_PLACEMENT_3D('',#7704,#6144,#6145);
#5325=AXIS2_PLACEMENT_3D('',#7707,#6147,#6148);
#5326=AXIS2_PLACEMENT_3D('',#7708,#6149,#6150);
#5327=AXIS2_PLACEMENT_3D('',#7710,#6151,#6152);
#5328=AXIS2_PLACEMENT_3D('',#7713,#6154,#6155);
#5329=AXIS2_PLACEMENT_3D('',#7714,#6156,#6157);
#5330=AXIS2_PLACEMENT_3D('',#7716,#6158,#6159);
#5331=AXIS2_PLACEMENT_3D('',#7719,#6161,#6162);
#5332=AXIS2_PLACEMENT_3D('',#7720,#6163,#6164);
#5333=AXIS2_PLACEMENT_3D('',#7722,#6165,#6166);
#5334=AXIS2_PLACEMENT_3D('',#7725,#6168,#6169);
#5335=AXIS2_PLACEMENT_3D('',#7726,#6170,#6171);
#5336=AXIS2_PLACEMENT_3D('',#7729,#6174,#6175);
#5337=AXIS2_PLACEMENT_3D('',#7738,#6180,#6181);
#5338=AXIS2_PLACEMENT_3D('',#7740,#6182,#6183);
#5339=AXIS2_PLACEMENT_3D('',#7743,#6185,#6186);
#5340=AXIS2_PLACEMENT_3D('',#7744,#6187,#6188);
#5341=AXIS2_PLACEMENT_3D('',#7746,#6189,#6190);
#5342=AXIS2_PLACEMENT_3D('',#7749,#6192,#6193);
#5343=AXIS2_PLACEMENT_3D('',#7750,#6194,#6195);
#5344=AXIS2_PLACEMENT_3D('',#7759,#6200,#6201);
#5345=AXIS2_PLACEMENT_3D('',#7768,#6206,#6207);
#5346=AXIS2_PLACEMENT_3D('',#7770,#6208,#6209);
#5347=AXIS2_PLACEMENT_3D('',#7773,#6211,#6212);
#5348=AXIS2_PLACEMENT_3D('',#7774,#6213,#6214);
#5349=AXIS2_PLACEMENT_3D('',#7776,#6215,#6216);
#5350=AXIS2_PLACEMENT_3D('',#7779,#6218,#6219);
#5351=AXIS2_PLACEMENT_3D('',#7780,#6220,#6221);
#5352=AXIS2_PLACEMENT_3D('',#7782,#6222,#6223);
#5353=AXIS2_PLACEMENT_3D('',#7785,#6225,#6226);
#5354=AXIS2_PLACEMENT_3D('',#7786,#6227,#6228);
#5355=AXIS2_PLACEMENT_3D('',#7788,#6229,#6230);
#5356=AXIS2_PLACEMENT_3D('',#7791,#6232,#6233);
#5357=AXIS2_PLACEMENT_3D('',#7792,#6234,#6235);
#5358=AXIS2_PLACEMENT_3D('',#7801,#6240,#6241);
#5359=AXIS2_PLACEMENT_3D('',#7810,#6246,#6247);
#5360=AXIS2_PLACEMENT_3D('',#7812,#6248,#6249);
#5361=AXIS2_PLACEMENT_3D('',#7815,#6251,#6252);
#5362=AXIS2_PLACEMENT_3D('',#7816,#6253,#6254);
#5363=AXIS2_PLACEMENT_3D('',#7818,#6255,#6256);
#5364=AXIS2_PLACEMENT_3D('',#7821,#6258,#6259);
#5365=AXIS2_PLACEMENT_3D('',#7822,#6260,#6261);
#5366=AXIS2_PLACEMENT_3D('',#7824,#6262,#6263);
#5367=AXIS2_PLACEMENT_3D('',#7827,#6265,#6266);
#5368=AXIS2_PLACEMENT_3D('',#7828,#6267,#6268);
#5369=AXIS2_PLACEMENT_3D('',#7830,#6269,#6270);
#5370=AXIS2_PLACEMENT_3D('',#7833,#6272,#6273);
#5371=AXIS2_PLACEMENT_3D('',#7834,#6274,#6275);
#5372=AXIS2_PLACEMENT_3D('',#7837,#6278,#6279);
#5373=AXIS2_PLACEMENT_3D('',#7846,#6284,#6285);
#5374=AXIS2_PLACEMENT_3D('',#7848,#6286,#6287);
#5375=AXIS2_PLACEMENT_3D('',#7851,#6289,#6290);
#5376=AXIS2_PLACEMENT_3D('',#7852,#6291,#6292);
#5377=AXIS2_PLACEMENT_3D('',#7854,#6293,#6294);
#5378=AXIS2_PLACEMENT_3D('',#7857,#6296,#6297);
#5379=AXIS2_PLACEMENT_3D('',#7858,#6298,#6299);
#5380=AXIS2_PLACEMENT_3D('',#7861,#6302,#6303);
#5381=AXIS2_PLACEMENT_3D('',#7864,#6306,#6307);
#5382=AXIS2_PLACEMENT_3D('',#7867,#6310,#6311);
#5383=AXIS2_PLACEMENT_3D('',#7876,#6316,#6317);
#5384=AXIS2_PLACEMENT_3D('',#7878,#6318,#6319);
#5385=AXIS2_PLACEMENT_3D('',#7881,#6321,#6322);
#5386=AXIS2_PLACEMENT_3D('',#7882,#6323,#6324);
#5387=AXIS2_PLACEMENT_3D('',#7884,#6325,#6326);
#5388=AXIS2_PLACEMENT_3D('',#7887,#6328,#6329);
#5389=AXIS2_PLACEMENT_3D('',#7888,#6330,#6331);
#5390=AXIS2_PLACEMENT_3D('',#7891,#6334,#6335);
#5391=AXIS2_PLACEMENT_3D('',#7894,#6338,#6339);
#5392=AXIS2_PLACEMENT_3D('',#7903,#6344,#6345);
#5393=AXIS2_PLACEMENT_3D('',#7909,#6349,#6350);
#5394=AXIS2_PLACEMENT_3D('',#7915,#6354,#6355);
#5395=AXIS2_PLACEMENT_3D('',#7917,#6356,#6357);
#5396=AXIS2_PLACEMENT_3D('',#7920,#6359,#6360);
#5397=AXIS2_PLACEMENT_3D('',#7921,#6361,#6362);
#5398=AXIS2_PLACEMENT_3D('',#7923,#6363,#6364);
#5399=AXIS2_PLACEMENT_3D('',#7926,#6366,#6367);
#5400=AXIS2_PLACEMENT_3D('',#7927,#6368,#6369);
#5401=AXIS2_PLACEMENT_3D('',#7933,#6373,#6374);
#5402=AXIS2_PLACEMENT_3D('',#7939,#6378,#6379);
#5403=AXIS2_PLACEMENT_3D('',#7945,#6383,#6384);
#5404=AXIS2_PLACEMENT_3D('',#7947,#6385,#6386);
#5405=AXIS2_PLACEMENT_3D('',#7950,#6388,#6389);
#5406=AXIS2_PLACEMENT_3D('',#7951,#6390,#6391);
#5407=AXIS2_PLACEMENT_3D('',#7960,#6396,#6397);
#5408=AXIS2_PLACEMENT_3D('',#7966,#6401,#6402);
#5409=AXIS2_PLACEMENT_3D('',#7972,#6406,#6407);
#5410=AXIS2_PLACEMENT_3D('',#7974,#6408,#6409);
#5411=AXIS2_PLACEMENT_3D('',#7977,#6411,#6412);
#5412=AXIS2_PLACEMENT_3D('',#7978,#6413,#6414);
#5413=AXIS2_PLACEMENT_3D('',#7980,#6415,#6416);
#5414=AXIS2_PLACEMENT_3D('',#7983,#6418,#6419);
#5415=AXIS2_PLACEMENT_3D('',#7984,#6420,#6421);
#5416=AXIS2_PLACEMENT_3D('',#7993,#6426,#6427);
#5417=AXIS2_PLACEMENT_3D('',#7999,#6431,#6432);
#5418=AXIS2_PLACEMENT_3D('',#8005,#6436,#6437);
#5419=AXIS2_PLACEMENT_3D('',#8007,#6438,#6439);
#5420=AXIS2_PLACEMENT_3D('',#8010,#6441,#6442);
#5421=AXIS2_PLACEMENT_3D('',#8011,#6443,#6444);
#5422=AXIS2_PLACEMENT_3D('',#8013,#6445,#6446);
#5423=AXIS2_PLACEMENT_3D('',#8016,#6448,#6449);
#5424=AXIS2_PLACEMENT_3D('',#8017,#6450,#6451);
#5425=AXIS2_PLACEMENT_3D('',#8023,#6455,#6456);
#5426=AXIS2_PLACEMENT_3D('',#8029,#6460,#6461);
#5427=AXIS2_PLACEMENT_3D('',#8032,#6464,#6465);
#5428=AXIS2_PLACEMENT_3D('',#8038,#6469,#6470);
#5429=AXIS2_PLACEMENT_3D('',#8044,#6474,#6475);
#5430=AXIS2_PLACEMENT_3D('',#8047,#6478,#6479);
#5431=AXIS2_PLACEMENT_3D('',#8053,#6483,#6484);
#5432=AXIS2_PLACEMENT_3D('',#8059,#6488,#6489);
#5433=AXIS2_PLACEMENT_3D('',#8062,#6492,#6493);
#5434=AXIS2_PLACEMENT_3D('',#8068,#6497,#6498);
#5435=AXIS2_PLACEMENT_3D('',#8074,#6502,#6503);
#5436=AXIS2_PLACEMENT_3D('',#8080,#6507,#6508);
#5437=AXIS2_PLACEMENT_3D('',#8082,#6509,#6510);
#5438=AXIS2_PLACEMENT_3D('',#8085,#6512,#6513);
#5439=AXIS2_PLACEMENT_3D('',#8086,#6514,#6515);
#5440=AXIS2_PLACEMENT_3D('',#8089,#6518,#6519);
#5441=AXIS2_PLACEMENT_3D('',#8098,#6524,#6525);
#5442=AXIS2_PLACEMENT_3D('',#8100,#6526,#6527);
#5443=AXIS2_PLACEMENT_3D('',#8103,#6529,#6530);
#5444=AXIS2_PLACEMENT_3D('',#8104,#6531,#6532);
#5445=AXIS2_PLACEMENT_3D('',#8106,#6533,#6534);
#5446=AXIS2_PLACEMENT_3D('',#8109,#6536,#6537);
#5447=AXIS2_PLACEMENT_3D('',#8110,#6538,#6539);
#5448=AXIS2_PLACEMENT_3D('',#8119,#6544,#6545);
#5449=AXIS2_PLACEMENT_3D('',#8122,#6548,#6549);
#5450=AXIS2_PLACEMENT_3D('',#8124,#6550,#6551);
#5451=AXIS2_PLACEMENT_3D('',#8127,#6553,#6554);
#5452=AXIS2_PLACEMENT_3D('',#8128,#6555,#6556);
#5453=AXIS2_PLACEMENT_3D('',#8130,#6557,#6558);
#5454=AXIS2_PLACEMENT_3D('',#8133,#6560,#6561);
#5455=AXIS2_PLACEMENT_3D('',#8134,#6562,#6563);
#5456=AXIS2_PLACEMENT_3D('',#8137,#6566,#6567);
#5457=AXIS2_PLACEMENT_3D('',#8140,#6570,#6571);
#5458=AXIS2_PLACEMENT_3D('',#8149,#6576,#6577);
#5459=AXIS2_PLACEMENT_3D('',#8155,#6581,#6582);
#5460=AXIS2_PLACEMENT_3D('',#8161,#6586,#6587);
#5461=AXIS2_PLACEMENT_3D('',#8163,#6588,#6589);
#5462=AXIS2_PLACEMENT_3D('',#8166,#6591,#6592);
#5463=AXIS2_PLACEMENT_3D('',#8167,#6593,#6594);
#5464=AXIS2_PLACEMENT_3D('',#8169,#6595,#6596);
#5465=AXIS2_PLACEMENT_3D('',#8172,#6598,#6599);
#5466=AXIS2_PLACEMENT_3D('',#8173,#6600,#6601);
#5467=AXIS2_PLACEMENT_3D('',#8179,#6605,#6606);
#5468=AXIS2_PLACEMENT_3D('',#8185,#6610,#6611);
#5469=AXIS2_PLACEMENT_3D('',#8191,#6615,#6616);
#5470=AXIS2_PLACEMENT_3D('',#8193,#6617,#6618);
#5471=AXIS2_PLACEMENT_3D('',#8196,#6620,#6621);
#5472=AXIS2_PLACEMENT_3D('',#8197,#6622,#6623);
#5473=AXIS2_PLACEMENT_3D('',#8206,#6628,#6629);
#5474=AXIS2_PLACEMENT_3D('',#8212,#6633,#6634);
#5475=AXIS2_PLACEMENT_3D('',#8218,#6638,#6639);
#5476=AXIS2_PLACEMENT_3D('',#8220,#6640,#6641);
#5477=AXIS2_PLACEMENT_3D('',#8223,#6643,#6644);
#5478=AXIS2_PLACEMENT_3D('',#8224,#6645,#6646);
#5479=AXIS2_PLACEMENT_3D('',#8226,#6647,#6648);
#5480=AXIS2_PLACEMENT_3D('',#8229,#6650,#6651);
#5481=AXIS2_PLACEMENT_3D('',#8230,#6652,#6653);
#5482=AXIS2_PLACEMENT_3D('',#8236,#6657,#6658);
#5483=AXIS2_PLACEMENT_3D('',#8242,#6662,#6663);
#5484=AXIS2_PLACEMENT_3D('',#8248,#6667,#6668);
#5485=AXIS2_PLACEMENT_3D('',#8250,#6669,#6670);
#5486=AXIS2_PLACEMENT_3D('',#8253,#6672,#6673);
#5487=AXIS2_PLACEMENT_3D('',#8254,#6674,#6675);
#5488=AXIS2_PLACEMENT_3D('',#8260,#6679,#6680);
#5489=AXIS2_PLACEMENT_3D('',#8266,#6684,#6685);
#5490=AXIS2_PLACEMENT_3D('',#8272,#6689,#6690);
#5491=AXIS2_PLACEMENT_3D('',#8274,#6691,#6692);
#5492=AXIS2_PLACEMENT_3D('',#8277,#6694,#6695);
#5493=AXIS2_PLACEMENT_3D('',#8278,#6696,#6697);
#5494=AXIS2_PLACEMENT_3D('',#8284,#6701,#6702);
#5495=AXIS2_PLACEMENT_3D('',#8290,#6706,#6707);
#5496=AXIS2_PLACEMENT_3D('',#8293,#6710,#6711);
#5497=AXIS2_PLACEMENT_3D('',#8299,#6715,#6716);
#5498=AXIS2_PLACEMENT_3D('',#8305,#6720,#6721);
#5499=AXIS2_PLACEMENT_3D('',#8308,#6724,#6725);
#5500=AXIS2_PLACEMENT_3D('',#8314,#6729,#6730);
#5501=AXIS2_PLACEMENT_3D('',#8320,#6734,#6735);
#5502=AXIS2_PLACEMENT_3D('',#8323,#6738,#6739);
#5503=AXIS2_PLACEMENT_3D('',#8326,#6742,#6743);
#5504=AXIS2_PLACEMENT_3D('',#8329,#6746,#6747);
#5505=AXIS2_PLACEMENT_3D('',#8331,#6748,#6749);
#5506=AXIS2_PLACEMENT_3D('',#8334,#6751,#6752);
#5507=AXIS2_PLACEMENT_3D('',#8335,#6753,#6754);
#5508=AXIS2_PLACEMENT_3D('',#8336,#6755,#6756);
#5724=DIRECTION('axis',(0.,0.,1.));
#5725=DIRECTION('refdir',(1.,0.,0.));
#5726=DIRECTION('center_axis',(-0.169919004238536,0.,0.985458031576477));
#5727=DIRECTION('ref_axis',(-0.985458031576477,0.,-0.169919004238536));
#5728=DIRECTION('',(0.985458031576477,0.,0.169919004238536));
#5729=DIRECTION('',(0.,1.,0.));
#5730=DIRECTION('',(-0.985458031576477,0.,-0.169919004238536));
#5731=DIRECTION('',(0.,-1.,0.));
#5732=DIRECTION('center_axis',(0.947303919134588,0.,0.320336205871659));
#5733=DIRECTION('ref_axis',(-0.320336205871659,0.,0.947303919134588));
#5734=DIRECTION('',(0.320336205871659,0.,-0.947303919134588));
#5735=DIRECTION('',(-0.320336205871659,0.,0.947303919134588));
#5736=DIRECTION('',(0.,-1.,0.));
#5737=DIRECTION('center_axis',(0.474184356164994,0.,-0.880425576848146));
#5738=DIRECTION('ref_axis',(0.880425576848146,0.,0.474184356164994));
#5739=DIRECTION('',(-0.880425576848146,0.,-0.474184356164994));
#5740=DIRECTION('',(0.880425576848146,0.,0.474184356164994));
#5741=DIRECTION('',(0.,-1.,0.));
#5742=DIRECTION('center_axis',(0.,-1.,0.));
#5743=DIRECTION('ref_axis',(1.,0.,0.));
#5744=DIRECTION('center_axis',(0.,1.,0.));
#5745=DIRECTION('ref_axis',(1.,0.,0.));
#5746=DIRECTION('',(0.,-1.,0.));
#5747=DIRECTION('center_axis',(0.,-1.,0.));
#5748=DIRECTION('ref_axis',(1.,0.,0.));
#5749=DIRECTION('center_axis',(0.,-1.,0.));
#5750=DIRECTION('ref_axis',(1.,0.,0.));
#5751=DIRECTION('center_axis',(0.,-1.,0.));
#5752=DIRECTION('ref_axis',(1.,0.,0.));
#5753=DIRECTION('',(0.,1.,0.));
#5754=DIRECTION('center_axis',(0.,1.,0.));
#5755=DIRECTION('ref_axis',(1.,0.,0.));
#5756=DIRECTION('center_axis',(0.441770335617579,0.,0.897128179564287));
#5757=DIRECTION('ref_axis',(-0.897128179564287,0.,0.441770335617579));
#5758=DIRECTION('',(0.897128179564287,0.,-0.441770335617579));
#5759=DIRECTION('',(0.,1.,0.));
#5760=DIRECTION('',(-0.897128179564287,0.,0.441770335617579));
#5761=DIRECTION('',(0.,-1.,0.));
#5762=DIRECTION('center_axis',(0.95467386700456,0.,-0.297653838642408));
#5763=DIRECTION('ref_axis',(0.297653838642408,0.,0.95467386700456));
#5764=DIRECTION('',(-0.297653838642408,0.,-0.95467386700456));
#5765=DIRECTION('',(0.297653838642408,0.,0.95467386700456));
#5766=DIRECTION('',(0.,-1.,0.));
#5767=DIRECTION('center_axis',(-0.13387796720821,0.,-0.990997825374101));
#5768=DIRECTION('ref_axis',(0.990997825374101,0.,-0.13387796720821));
#5769=DIRECTION('',(-0.990997825374101,0.,0.13387796720821));
#5770=DIRECTION('',(0.990997825374101,0.,-0.13387796720821));
#5771=DIRECTION('',(0.,-1.,0.));
#5772=DIRECTION('center_axis',(0.,-1.,0.));
#5773=DIRECTION('ref_axis',(1.,0.,0.));
#5774=DIRECTION('center_axis',(0.,1.,0.));
#5775=DIRECTION('ref_axis',(1.,0.,0.));
#5776=DIRECTION('',(0.,-1.,0.));
#5777=DIRECTION('center_axis',(0.,-1.,0.));
#5778=DIRECTION('ref_axis',(1.,0.,0.));
#5779=DIRECTION('center_axis',(0.,-1.,0.));
#5780=DIRECTION('ref_axis',(1.,0.,0.));
#5781=DIRECTION('center_axis',(0.,-1.,0.));
#5782=DIRECTION('ref_axis',(1.,0.,0.));
#5783=DIRECTION('',(0.,1.,0.));
#5784=DIRECTION('center_axis',(0.,1.,0.));
#5785=DIRECTION('ref_axis',(1.,0.,0.));
#5786=DIRECTION('center_axis',(0.0386823792600046,0.,0.999251556683694));
#5787=DIRECTION('ref_axis',(-0.999251556683694,0.,0.0386823792600046));
#5788=DIRECTION('',(0.999251556683694,0.,-0.0386823792600046));
#5789=DIRECTION('',(-0.999251556683694,0.,0.0386823792600046));
#5790=DIRECTION('',(0.,-1.,0.));
#5791=DIRECTION('center_axis',(0.993204697860151,0.,0.116380531655973));
#5792=DIRECTION('ref_axis',(-0.116380531655973,0.,0.993204697860151));
#5793=DIRECTION('',(0.116380531655973,0.,-0.993204697860151));
#5794=DIRECTION('',(-0.116380531655973,0.,0.993204697860151));
#5795=DIRECTION('',(0.,-1.,0.));
#5796=DIRECTION('center_axis',(0.280771519966595,0.,-0.959774636868285));
#5797=DIRECTION('ref_axis',(0.959774636868285,0.,0.280771519966595));
#5798=DIRECTION('',(-0.959774636868285,0.,-0.280771519966595));
#5799=DIRECTION('',(0.959774636868285,0.,0.280771519966595));
#5800=DIRECTION('',(0.,-1.,0.));
#5801=DIRECTION('center_axis',(0.,-1.,0.));
#5802=DIRECTION('ref_axis',(1.,0.,0.));
#5803=DIRECTION('center_axis',(0.,-1.,0.));
#5804=DIRECTION('ref_axis',(1.,0.,0.));
#5805=DIRECTION('',(0.,1.,0.));
#5806=DIRECTION('center_axis',(0.,1.,0.));
#5807=DIRECTION('ref_axis',(1.,0.,0.));
#5808=DIRECTION('center_axis',(0.884718422489227,0.,0.466125855223859));
#5809=DIRECTION('ref_axis',(-0.466125855223859,0.,0.884718422489227));
#5810=DIRECTION('',(0.466125855223858,0.,-0.884718422489227));
#5811=DIRECTION('',(0.,1.,0.));
#5812=DIRECTION('',(-0.466125855223858,0.,0.884718422489227));
#5813=DIRECTION('',(0.,-1.,0.));
#5814=DIRECTION('center_axis',(0.597390845850087,0.,-0.801950233676952));
#5815=DIRECTION('ref_axis',(0.801950233676952,0.,0.597390845850087));
#5816=DIRECTION('',(-0.801950233676952,0.,-0.597390845850087));
#5817=DIRECTION('',(0.801950233676952,0.,0.597390845850087));
#5818=DIRECTION('',(0.,-1.,0.));
#5819=DIRECTION('center_axis',(-0.690803457452622,0.,-0.723042587384383));
#5820=DIRECTION('ref_axis',(0.723042587384383,0.,-0.690803457452622));
#5821=DIRECTION('',(-0.723042587384383,0.,0.690803457452622));
#5822=DIRECTION('',(0.723042587384383,0.,-0.690803457452622));
#5823=DIRECTION('',(0.,-1.,0.));
#5824=DIRECTION('center_axis',(0.,-1.,0.));
#5825=DIRECTION('ref_axis',(1.,0.,0.));
#5826=DIRECTION('center_axis',(0.,1.,0.));
#5827=DIRECTION('ref_axis',(1.,0.,0.));
#5828=DIRECTION('',(0.,-1.,0.));
#5829=DIRECTION('center_axis',(0.,-1.,0.));
#5830=DIRECTION('ref_axis',(1.,0.,0.));
#5831=DIRECTION('center_axis',(0.,-1.,0.));
#5832=DIRECTION('ref_axis',(1.,0.,0.));
#5833=DIRECTION('center_axis',(0.,-1.,0.));
#5834=DIRECTION('ref_axis',(1.,0.,0.));
#5835=DIRECTION('',(0.,1.,0.));
#5836=DIRECTION('center_axis',(0.,1.,0.));
#5837=DIRECTION('ref_axis',(1.,0.,0.));
#5838=DIRECTION('center_axis',(0.245593157166234,0.,0.969372993822874));
#5839=DIRECTION('ref_axis',(-0.969372993822874,0.,0.245593157166234));
#5840=DIRECTION('',(0.969372993822874,0.,-0.245593157166234));
#5841=DIRECTION('',(-0.969372993822874,0.,0.245593157166234));
#5842=DIRECTION('',(0.,-1.,0.));
#5843=DIRECTION('center_axis',(0.995697665364314,0.,-0.0926615302488318));
#5844=DIRECTION('ref_axis',(0.0926615302488318,0.,0.995697665364314));
#5845=DIRECTION('',(-0.0926615302488317,0.,-0.995697665364314));
#5846=DIRECTION('',(0.0926615302488317,0.,0.995697665364314));
#5847=DIRECTION('',(0.,-1.,0.));
#5848=DIRECTION('center_axis',(0.075087621054422,0.,-0.997176939747599));
#5849=DIRECTION('ref_axis',(0.997176939747599,0.,0.075087621054422));
#5850=DIRECTION('',(-0.997176939747599,0.,-0.075087621054422));
#5851=DIRECTION('',(0.997176939747599,0.,0.075087621054422));
#5852=DIRECTION('center_axis',(0.618640030553172,0.,0.785674558960115));
#5853=DIRECTION('ref_axis',(-0.785674558960115,0.,0.618640030553172));
#5854=DIRECTION('',(0.785674558960114,0.,-0.618640030553172));
#5855=DIRECTION('',(-0.785674558960115,0.,0.618640030553172));
#5856=DIRECTION('',(0.,-1.,0.));
#5857=DIRECTION('center_axis',(0.871926239623235,0.,-0.489637245985725));
#5858=DIRECTION('ref_axis',(0.489637245985725,0.,0.871926239623235));
#5859=DIRECTION('',(-0.489637245985725,0.,-0.871926239623235));
#5860=DIRECTION('',(0.489637245985725,0.,0.871926239623235));
#5861=DIRECTION('',(0.,-1.,0.));
#5862=DIRECTION('center_axis',(-0.336992445886082,0.,-0.941507350696592));
#5863=DIRECTION('ref_axis',(0.941507350696592,0.,-0.336992445886082));
#5864=DIRECTION('',(-0.941507350696592,0.,0.336992445886082));
#5865=DIRECTION('',(0.941507350696592,0.,-0.336992445886082));
#5866=DIRECTION('',(0.,-1.,0.));
#5867=DIRECTION('center_axis',(0.,-1.,0.));
#5868=DIRECTION('ref_axis',(1.,0.,0.));
#5869=DIRECTION('center_axis',(0.,-1.,0.));
#5870=DIRECTION('ref_axis',(1.,0.,0.));
#5871=DIRECTION('',(0.,1.,0.));
#5872=DIRECTION('center_axis',(0.,1.,0.));
#5873=DIRECTION('ref_axis',(1.,0.,0.));
#5874=DIRECTION('center_axis',(-0.371094111890007,0.,0.928595261737086));
#5875=DIRECTION('ref_axis',(-0.928595261737086,0.,-0.371094111890007));
#5876=DIRECTION('',(0.928595261737086,0.,0.371094111890007));
#5877=DIRECTION('',(0.,1.,0.));
#5878=DIRECTION('',(-0.928595261737086,0.,-0.371094111890007));
#5879=DIRECTION('',(0.,-1.,0.));
#5880=DIRECTION('center_axis',(0.860001413474306,0.,0.510291650747096));
#5881=DIRECTION('ref_axis',(-0.510291650747096,0.,0.860001413474306));
#5882=DIRECTION('',(0.510291650747096,0.,-0.860001413474306));
#5883=DIRECTION('',(-0.510291650747096,0.,0.860001413474306));
#5884=DIRECTION('',(0.,-1.,0.));
#5885=DIRECTION('center_axis',(0.646873060609993,0.,-0.762597694369096));
#5886=DIRECTION('ref_axis',(0.762597694369096,0.,0.646873060609993));
#5887=DIRECTION('',(-0.762597694369096,0.,-0.646873060609993));
#5888=DIRECTION('',(0.762597694369096,0.,0.646873060609993));
#5889=DIRECTION('center_axis',(0.,-1.,0.));
#5890=DIRECTION('ref_axis',(1.,0.,0.));
#5891=DIRECTION('center_axis',(0.,1.,0.));
#5892=DIRECTION('ref_axis',(1.,0.,0.));
#5893=DIRECTION('',(0.,-1.,0.));
#5894=DIRECTION('center_axis',(0.,-1.,0.));
#5895=DIRECTION('ref_axis',(1.,0.,0.));
#5896=DIRECTION('center_axis',(0.768472187589369,0.,0.639883190044566));
#5897=DIRECTION('ref_axis',(-0.639883190044566,0.,0.768472187589369));
#5898=DIRECTION('',(0.639883190044566,0.,-0.768472187589369));
#5899=DIRECTION('',(-0.639883190044566,0.,0.768472187589368));
#5900=DIRECTION('',(0.,-1.,0.));
#5901=DIRECTION('center_axis',(0.751071251604073,0.,-0.660221156139283));
#5902=DIRECTION('ref_axis',(0.660221156139283,0.,0.751071251604073));
#5903=DIRECTION('',(-0.660221156139283,0.,-0.751071251604073));
#5904=DIRECTION('',(0.660221156139283,0.,0.751071251604073));
#5905=DIRECTION('',(0.,-1.,0.));
#5906=DIRECTION('center_axis',(-0.525378737609566,0.,-0.850868486940126));
#5907=DIRECTION('ref_axis',(0.850868486940126,0.,-0.525378737609566));
#5908=DIRECTION('',(-0.850868486940126,0.,0.525378737609565));
#5909=DIRECTION('',(0.850868486940126,0.,-0.525378737609565));
#5910=DIRECTION('center_axis',(-0.743144825477394,0.,-0.669130606358858));
#5911=DIRECTION('ref_axis',(0.669130606358858,0.,-0.743144825477394));
#5912=DIRECTION('',(-0.669130606358858,0.,0.743144825477394));
#5913=DIRECTION('',(0.,1.,0.));
#5914=DIRECTION('',(0.669130606358858,0.,-0.743144825477394));
#5915=DIRECTION('',(0.,-1.,0.));
#5916=DIRECTION('center_axis',(0.743144825477394,0.,0.669130606358858));
#5917=DIRECTION('ref_axis',(-0.669130606358858,0.,0.743144825477394));
#5918=DIRECTION('',(0.669130606358858,0.,-0.743144825477394));
#5919=DIRECTION('',(0.,1.,0.));
#5920=DIRECTION('',(-0.669130606358858,0.,0.743144825477394));
#5921=DIRECTION('',(0.,-1.,0.));
#5922=DIRECTION('center_axis',(0.,-1.,0.));
#5923=DIRECTION('ref_axis',(1.,0.,0.));
#5924=DIRECTION('center_axis',(0.,-1.,0.));
#5925=DIRECTION('ref_axis',(1.,0.,0.));
#5926=DIRECTION('',(0.,-1.,0.));
#5927=DIRECTION('center_axis',(0.,1.,0.));
#5928=DIRECTION('ref_axis',(1.,0.,0.));
#5929=DIRECTION('center_axis',(0.,-1.,0.));
#5930=DIRECTION('ref_axis',(1.,0.,0.));
#5931=DIRECTION('center_axis',(0.,1.,0.));
#5932=DIRECTION('ref_axis',(1.,0.,0.));
#5933=DIRECTION('',(0.,1.,0.));
#5934=DIRECTION('center_axis',(0.,-1.,0.));
#5935=DIRECTION('ref_axis',(1.,0.,0.));
#5936=DIRECTION('center_axis',(0.,-1.,0.));
#5937=DIRECTION('ref_axis',(1.,0.,0.));
#5938=DIRECTION('center_axis',(0.,-1.,0.));
#5939=DIRECTION('ref_axis',(1.,0.,0.));
#5940=DIRECTION('',(0.,1.,0.));
#5941=DIRECTION('center_axis',(0.,1.,0.));
#5942=DIRECTION('ref_axis',(1.,0.,0.));
#5943=DIRECTION('center_axis',(0.,-1.,0.));
#5944=DIRECTION('ref_axis',(1.,0.,0.));
#5945=DIRECTION('center_axis',(0.,1.,0.));
#5946=DIRECTION('ref_axis',(1.,0.,0.));
#5947=DIRECTION('',(0.,-1.,0.));
#5948=DIRECTION('center_axis',(0.,-1.,0.));
#5949=DIRECTION('ref_axis',(1.,0.,0.));
#5950=DIRECTION('center_axis',(-0.4067366430758,0.,-0.913545457642601));
#5951=DIRECTION('ref_axis',(0.913545457642601,0.,-0.4067366430758));
#5952=DIRECTION('',(-0.913545457642601,0.,0.4067366430758));
#5953=DIRECTION('',(0.913545457642601,0.,-0.4067366430758));
#5954=DIRECTION('center_axis',(0.4067366430758,0.,0.913545457642601));
#5955=DIRECTION('ref_axis',(-0.913545457642601,0.,0.4067366430758));
#5956=DIRECTION('',(0.913545457642601,0.,-0.4067366430758));
#5957=DIRECTION('',(0.,1.,0.));
#5958=DIRECTION('',(-0.913545457642601,0.,0.4067366430758));
#5959=DIRECTION('',(0.,-1.,0.));
#5960=DIRECTION('center_axis',(0.,-1.,0.));
#5961=DIRECTION('ref_axis',(1.,0.,0.));
#5962=DIRECTION('center_axis',(0.,1.,0.));
#5963=DIRECTION('ref_axis',(1.,0.,0.));
#5964=DIRECTION('',(0.,1.,0.));
#5965=DIRECTION('center_axis',(0.,-1.,0.));
#5966=DIRECTION('ref_axis',(1.,0.,0.));
#5967=DIRECTION('center_axis',(0.,-1.,0.));
#5968=DIRECTION('ref_axis',(1.,0.,0.));
#5969=DIRECTION('center_axis',(0.,1.,0.));
#5970=DIRECTION('ref_axis',(1.,0.,0.));
#5971=DIRECTION('',(0.,-1.,0.));
#5972=DIRECTION('center_axis',(0.,-1.,0.));
#5973=DIRECTION('ref_axis',(1.,0.,0.));
#5974=DIRECTION('center_axis',(-0.951056516295154,0.,-0.309016994374948));
#5975=DIRECTION('ref_axis',(0.309016994374948,0.,-0.951056516295154));
#5976=DIRECTION('',(-0.309016994374948,0.,0.951056516295154));
#5977=DIRECTION('',(0.,1.,0.));
#5978=DIRECTION('',(0.309016994374948,0.,-0.951056516295154));
#5979=DIRECTION('',(0.,-1.,0.));
#5980=DIRECTION('center_axis',(0.951056516295154,0.,0.309016994374948));
#5981=DIRECTION('ref_axis',(-0.309016994374948,0.,0.951056516295154));
#5982=DIRECTION('',(0.309016994374948,0.,-0.951056516295154));
#5983=DIRECTION('',(-0.309016994374948,0.,0.951056516295154));
#5984=DIRECTION('center_axis',(0.,-1.,0.));
#5985=DIRECTION('ref_axis',(1.,0.,0.));
#5986=DIRECTION('center_axis',(0.,-1.,0.));
#5987=DIRECTION('ref_axis',(1.,0.,0.));
#5988=DIRECTION('',(0.,-1.,0.));
#5989=DIRECTION('center_axis',(0.,1.,0.));
#5990=DIRECTION('ref_axis',(1.,0.,0.));
#5991=DIRECTION('center_axis',(0.,-1.,0.));
#5992=DIRECTION('ref_axis',(1.,0.,0.));
#5993=DIRECTION('center_axis',(0.,-1.,0.));
#5994=DIRECTION('ref_axis',(1.,0.,0.));
#5995=DIRECTION('',(0.,1.,0.));
#5996=DIRECTION('center_axis',(0.,1.,0.));
#5997=DIRECTION('ref_axis',(1.,0.,0.));
#5998=DIRECTION('center_axis',(-0.846036043229222,0.,0.533125701459836));
#5999=DIRECTION('ref_axis',(-0.533125701459836,0.,-0.846036043229222));
#6000=DIRECTION('',(0.533125701459836,0.,0.846036043229222));
#6001=DIRECTION('',(0.,1.,0.));
#6002=DIRECTION('',(-0.533125701459836,0.,-0.846036043229222));
#6003=DIRECTION('',(0.,-1.,0.));
#6004=DIRECTION('center_axis',(0.395813852010064,0.,0.918330765332925));
#6005=DIRECTION('ref_axis',(-0.918330765332925,0.,0.395813852010064));
#6006=DIRECTION('',(0.918330765332925,0.,-0.395813852010064));
#6007=DIRECTION('',(-0.918330765332925,0.,0.395813852010064));
#6008=DIRECTION('',(0.,-1.,0.));
#6009=DIRECTION('center_axis',(0.971574977419217,0.,-0.236732049483902));
#6010=DIRECTION('ref_axis',(0.236732049483902,0.,0.971574977419217));
#6011=DIRECTION('',(-0.236732049483902,0.,-0.971574977419217));
#6012=DIRECTION('',(0.236732049483902,0.,0.971574977419217));
#6013=DIRECTION('',(0.,-1.,0.));
#6014=DIRECTION('center_axis',(0.,-1.,0.));
#6015=DIRECTION('ref_axis',(1.,0.,0.));
#6016=DIRECTION('center_axis',(0.,1.,0.));
#6017=DIRECTION('ref_axis',(1.,0.,0.));
#6018=DIRECTION('',(0.,-1.,0.));
#6019=DIRECTION('center_axis',(0.,-1.,0.));
#6020=DIRECTION('ref_axis',(1.,0.,0.));
#6021=DIRECTION('center_axis',(0.,-1.,0.));
#6022=DIRECTION('ref_axis',(1.,0.,0.));
#6023=DIRECTION('center_axis',(0.,-1.,0.));
#6024=DIRECTION('ref_axis',(1.,0.,0.));
#6025=DIRECTION('',(0.,1.,0.));
#6026=DIRECTION('center_axis',(0.,1.,0.));
#6027=DIRECTION('ref_axis',(1.,0.,0.));
#6028=DIRECTION('center_axis',(-0.99782096176235,0.,-0.0659797564989425));
#6029=DIRECTION('ref_axis',(0.0659797564989425,0.,-0.99782096176235));
#6030=DIRECTION('',(-0.0659797564989425,0.,0.997820961762349));
#6031=DIRECTION('',(0.,1.,0.));
#6032=DIRECTION('',(0.0659797564989425,0.,-0.997820961762349));
#6033=DIRECTION('',(0.,-1.,0.));
#6034=DIRECTION('center_axis',(-0.219561147704,0.,0.975598740476279));
#6035=DIRECTION('ref_axis',(-0.975598740476279,0.,-0.219561147704));
#6036=DIRECTION('',(0.975598740476279,0.,0.219561147704));
#6037=DIRECTION('',(-0.975598740476279,0.,-0.219561147704));
#6038=DIRECTION('',(0.,-1.,0.));
#6039=DIRECTION('center_axis',(0.925168275473212,0.,0.37955719207772));
#6040=DIRECTION('ref_axis',(-0.37955719207772,0.,0.925168275473212));
#6041=DIRECTION('',(0.37955719207772,0.,-0.925168275473212));
#6042=DIRECTION('',(-0.37955719207772,0.,0.925168275473212));
#6043=DIRECTION('',(0.,-1.,0.));
#6044=DIRECTION('center_axis',(0.,-1.,0.));
#6045=DIRECTION('ref_axis',(1.,0.,0.));
#6046=DIRECTION('center_axis',(0.,1.,0.));
#6047=DIRECTION('ref_axis',(1.,0.,0.));
#6048=DIRECTION('',(0.,-1.,0.));
#6049=DIRECTION('center_axis',(0.,-1.,0.));
#6050=DIRECTION('ref_axis',(1.,0.,0.));
#6051=DIRECTION('center_axis',(0.,-1.,0.));
#6052=DIRECTION('ref_axis',(1.,0.,0.));
#6053=DIRECTION('center_axis',(0.,-1.,0.));
#6054=DIRECTION('ref_axis',(1.,0.,0.));
#6055=DIRECTION('',(0.,1.,0.));
#6056=DIRECTION('center_axis',(0.,1.,0.));
#6057=DIRECTION('ref_axis',(1.,0.,0.));
#6058=DIRECTION('center_axis',(-0.98973414244318,0.,0.142920702776972));
#6059=DIRECTION('ref_axis',(-0.142920702776972,0.,-0.98973414244318));
#6060=DIRECTION('',(0.142920702776972,0.,0.98973414244318));
#6061=DIRECTION('',(-0.142920702776972,0.,-0.98973414244318));
#6062=DIRECTION('',(0.,-1.,0.));
#6063=DIRECTION('center_axis',(-0.0119248261489288,0.,0.999928896732822));
#6064=DIRECTION('ref_axis',(-0.999928896732822,0.,-0.0119248261489288));
#6065=DIRECTION('',(0.999928896732822,0.,0.0119248261489288));
#6066=DIRECTION('',(-0.999928896732822,0.,-0.0119248261489288));
#6067=DIRECTION('',(0.,-1.,0.));
#6068=DIRECTION('center_axis',(0.983865506496075,0.,0.178909656327496));
#6069=DIRECTION('ref_axis',(-0.178909656327496,0.,0.983865506496075));
#6070=DIRECTION('',(0.178909656327496,0.,-0.983865506496075));
#6071=DIRECTION('',(-0.178909656327496,0.,0.983865506496075));
#6072=DIRECTION('',(0.,-1.,0.));
#6073=DIRECTION('center_axis',(0.,-1.,0.));
#6074=DIRECTION('ref_axis',(1.,0.,0.));
#6075=DIRECTION('center_axis',(0.,-1.,0.));
#6076=DIRECTION('ref_axis',(1.,0.,0.));
#6077=DIRECTION('',(0.,1.,0.));
#6078=DIRECTION('center_axis',(0.,1.,0.));
#6079=DIRECTION('ref_axis',(1.,0.,0.));
#6080=DIRECTION('center_axis',(-0.938391191827905,0.,0.34557484153191));
#6081=DIRECTION('ref_axis',(-0.34557484153191,0.,-0.938391191827905));
#6082=DIRECTION('',(0.34557484153191,0.,0.938391191827905));
#6083=DIRECTION('',(-0.34557484153191,0.,-0.938391191827905));
#6084=DIRECTION('',(0.,-1.,0.));
#6085=DIRECTION('center_axis',(0.196232667530515,0.,0.980557362010943));
#6086=DIRECTION('ref_axis',(-0.980557362010943,0.,0.196232667530515));
#6087=DIRECTION('',(0.980557362010942,0.,-0.196232667530515));
#6088=DIRECTION('',(-0.980557362010942,0.,0.196232667530515));
#6089=DIRECTION('',(0.,-1.,0.));
#6090=DIRECTION('center_axis',(0.99956309377456,0.,-0.0295570899080193));
#6091=DIRECTION('ref_axis',(0.0295570899080193,0.,0.99956309377456));
#6092=DIRECTION('',(-0.0295570899080193,0.,-0.99956309377456));
#6093=DIRECTION('',(0.0295570899080193,0.,0.99956309377456));
#6094=DIRECTION('center_axis',(-0.716705059810067,0.,0.69737641001302));
#6095=DIRECTION('ref_axis',(-0.69737641001302,0.,-0.716705059810067));
#6096=DIRECTION('',(0.69737641001302,0.,0.716705059810067));
#6097=DIRECTION('',(-0.69737641001302,0.,-0.716705059810067));
#6098=DIRECTION('',(0.,-1.,0.));
#6099=DIRECTION('center_axis',(0.578096071831186,0.,0.815968707569937));
#6100=DIRECTION('ref_axis',(-0.815968707569937,0.,0.578096071831186));
#6101=DIRECTION('',(0.815968707569936,0.,-0.578096071831186));
#6102=DIRECTION('',(-0.815968707569936,0.,0.578096071831186));
#6103=DIRECTION('',(0.,-1.,0.));
#6104=DIRECTION('center_axis',(0.901124372416657,0.,-0.433560682530931));
#6105=DIRECTION('ref_axis',(0.433560682530931,0.,0.901124372416657));
#6106=DIRECTION('',(-0.433560682530931,0.,-0.901124372416657));
#6107=DIRECTION('',(0.433560682530931,0.,0.901124372416657));
#6108=DIRECTION('',(0.,-1.,0.));
#6109=DIRECTION('center_axis',(0.,-1.,0.));
#6110=DIRECTION('ref_axis',(1.,0.,0.));
#6111=DIRECTION('center_axis',(0.,-1.,0.));
#6112=DIRECTION('ref_axis',(1.,0.,0.));
#6113=DIRECTION('',(0.,1.,0.));
#6114=DIRECTION('center_axis',(0.,1.,0.));
#6115=DIRECTION('ref_axis',(1.,0.,0.));
#6116=DIRECTION('center_axis',(-0.556050626144771,0.,0.831148423065344));
#6117=DIRECTION('ref_axis',(-0.831148423065344,0.,-0.556050626144771));
#6118=DIRECTION('',(0.831148423065344,0.,0.556050626144771));
#6119=DIRECTION('',(-0.831148423065344,0.,-0.556050626144771));
#6120=DIRECTION('',(0.,-1.,0.));
#6121=DIRECTION('center_axis',(0.735112719300559,0.,0.677944901833871));
#6122=DIRECTION('ref_axis',(-0.677944901833871,0.,0.735112719300559));
#6123=DIRECTION('',(0.677944901833871,0.,-0.735112719300559));
#6124=DIRECTION('',(-0.677944901833871,0.,0.735112719300559));
#6125=DIRECTION('',(0.,-1.,0.));
#6126=DIRECTION('center_axis',(0.791290308265002,0.,-0.61144063329638));
#6127=DIRECTION('ref_axis',(0.61144063329638,0.,0.791290308265002));
#6128=DIRECTION('',(-0.61144063329638,0.,-0.791290308265002));
#6129=DIRECTION('',(0.61144063329638,0.,0.791290308265002));
#6130=DIRECTION('center_axis',(0.866025403784438,0.,0.5));
#6131=DIRECTION('ref_axis',(-0.5,0.,0.866025403784438));
#6132=DIRECTION('',(0.5,0.,-0.866025403784438));
#6133=DIRECTION('',(0.,1.,0.));
#6134=DIRECTION('',(-0.5,0.,0.866025403784438));
#6135=DIRECTION('',(0.,-1.,0.));
#6136=DIRECTION('center_axis',(-0.866025403784438,0.,-0.5));
#6137=DIRECTION('ref_axis',(0.5,0.,-0.866025403784438));
#6138=DIRECTION('',(-0.5,0.,0.866025403784438));
#6139=DIRECTION('',(0.,1.,0.));
#6140=DIRECTION('',(0.5,0.,-0.866025403784438));
#6141=DIRECTION('',(0.,-1.,0.));
#6142=DIRECTION('center_axis',(0.,-1.,0.));
#6143=DIRECTION('ref_axis',(1.,0.,0.));
#6144=DIRECTION('center_axis',(0.,-1.,0.));
#6145=DIRECTION('ref_axis',(1.,0.,0.));
#6146=DIRECTION('',(0.,-1.,0.));
#6147=DIRECTION('center_axis',(0.,1.,0.));
#6148=DIRECTION('ref_axis',(1.,0.,0.));
#6149=DIRECTION('center_axis',(0.,-1.,0.));
#6150=DIRECTION('ref_axis',(1.,0.,0.));
#6151=DIRECTION('center_axis',(0.,1.,0.));
#6152=DIRECTION('ref_axis',(1.,0.,0.));
#6153=DIRECTION('',(0.,1.,0.));
#6154=DIRECTION('center_axis',(0.,-1.,0.));
#6155=DIRECTION('ref_axis',(1.,0.,0.));
#6156=DIRECTION('center_axis',(0.,-1.,0.));
#6157=DIRECTION('ref_axis',(1.,0.,0.));
#6158=DIRECTION('center_axis',(0.,-1.,0.));
#6159=DIRECTION('ref_axis',(1.,0.,0.));
#6160=DIRECTION('',(0.,1.,0.));
#6161=DIRECTION('center_axis',(0.,1.,0.));
#6162=DIRECTION('ref_axis',(1.,0.,0.));
#6163=DIRECTION('center_axis',(0.,-1.,0.));
#6164=DIRECTION('ref_axis',(1.,0.,0.));
#6165=DIRECTION('center_axis',(0.,1.,0.));
#6166=DIRECTION('ref_axis',(1.,0.,0.));
#6167=DIRECTION('',(0.,-1.,0.));
#6168=DIRECTION('center_axis',(0.,-1.,0.));
#6169=DIRECTION('ref_axis',(1.,0.,0.));
#6170=DIRECTION('center_axis',(0.587785252292473,0.,0.809016994374948));
#6171=DIRECTION('ref_axis',(-0.809016994374948,0.,0.587785252292473));
#6172=DIRECTION('',(0.809016994374947,0.,-0.587785252292473));
#6173=DIRECTION('',(-0.809016994374947,0.,0.587785252292473));
#6174=DIRECTION('center_axis',(-0.587785252292473,0.,-0.809016994374948));
#6175=DIRECTION('ref_axis',(0.809016994374948,0.,-0.587785252292473));
#6176=DIRECTION('',(-0.809016994374947,0.,0.587785252292473));
#6177=DIRECTION('',(0.,1.,0.));
#6178=DIRECTION('',(0.809016994374947,0.,-0.587785252292473));
#6179=DIRECTION('',(0.,-1.,0.));
#6180=DIRECTION('center_axis',(0.,-1.,0.));
#6181=DIRECTION('ref_axis',(1.,0.,0.));
#6182=DIRECTION('center_axis',(0.,1.,0.));
#6183=DIRECTION('ref_axis',(1.,0.,0.));
#6184=DIRECTION('',(0.,1.,0.));
#6185=DIRECTION('center_axis',(0.,-1.,0.));
#6186=DIRECTION('ref_axis',(1.,0.,0.));
#6187=DIRECTION('center_axis',(0.,-1.,0.));
#6188=DIRECTION('ref_axis',(1.,0.,0.));
#6189=DIRECTION('center_axis',(0.,1.,0.));
#6190=DIRECTION('ref_axis',(1.,0.,0.));
#6191=DIRECTION('',(0.,-1.,0.));
#6192=DIRECTION('center_axis',(0.,-1.,0.));
#6193=DIRECTION('ref_axis',(1.,0.,0.));
#6194=DIRECTION('center_axis',(0.951056516295154,0.,-0.309016994374947));
#6195=DIRECTION('ref_axis',(0.309016994374947,0.,0.951056516295154));
#6196=DIRECTION('',(-0.309016994374947,0.,-0.951056516295154));
#6197=DIRECTION('',(0.,1.,0.));
#6198=DIRECTION('',(0.309016994374947,0.,0.951056516295154));
#6199=DIRECTION('',(0.,-1.,0.));
#6200=DIRECTION('center_axis',(-0.951056516295154,0.,0.309016994374947));
#6201=DIRECTION('ref_axis',(-0.309016994374947,0.,-0.951056516295154));
#6202=DIRECTION('',(0.309016994374947,0.,0.951056516295154));
#6203=DIRECTION('',(0.,1.,0.));
#6204=DIRECTION('',(-0.309016994374947,0.,-0.951056516295154));
#6205=DIRECTION('',(0.,-1.,0.));
#6206=DIRECTION('center_axis',(0.,-1.,0.));
#6207=DIRECTION('ref_axis',(1.,0.,0.));
#6208=DIRECTION('center_axis',(0.,-1.,0.));
#6209=DIRECTION('ref_axis',(1.,0.,0.));
#6210=DIRECTION('',(0.,-1.,0.));
#6211=DIRECTION('center_axis',(0.,1.,0.));
#6212=DIRECTION('ref_axis',(1.,0.,0.));
#6213=DIRECTION('center_axis',(0.,-1.,0.));
#6214=DIRECTION('ref_axis',(1.,0.,0.));
#6215=DIRECTION('center_axis',(0.,1.,0.));
#6216=DIRECTION('ref_axis',(1.,0.,0.));
#6217=DIRECTION('',(0.,1.,0.));
#6218=DIRECTION('center_axis',(0.,-1.,0.));
#6219=DIRECTION('ref_axis',(1.,0.,0.));
#6220=DIRECTION('center_axis',(0.,-1.,0.));
#6221=DIRECTION('ref_axis',(1.,0.,0.));
#6222=DIRECTION('center_axis',(0.,-1.,0.));
#6223=DIRECTION('ref_axis',(1.,0.,0.));
#6224=DIRECTION('',(0.,1.,0.));
#6225=DIRECTION('center_axis',(0.,1.,0.));
#6226=DIRECTION('ref_axis',(1.,0.,0.));
#6227=DIRECTION('center_axis',(0.,-1.,0.));
#6228=DIRECTION('ref_axis',(1.,0.,0.));
#6229=DIRECTION('center_axis',(0.,1.,0.));
#6230=DIRECTION('ref_axis',(1.,0.,0.));
#6231=DIRECTION('',(0.,-1.,0.));
#6232=DIRECTION('center_axis',(0.,-1.,0.));
#6233=DIRECTION('ref_axis',(1.,0.,0.));
#6234=DIRECTION('center_axis',(0.406736643075801,0.,-0.913545457642601));
#6235=DIRECTION('ref_axis',(0.913545457642601,0.,0.406736643075801));
#6236=DIRECTION('',(-0.913545457642601,0.,-0.406736643075801));
#6237=DIRECTION('',(0.,1.,0.));
#6238=DIRECTION('',(0.913545457642601,0.,0.406736643075801));
#6239=DIRECTION('',(0.,-1.,0.));
#6240=DIRECTION('center_axis',(-0.406736643075801,0.,0.913545457642601));
#6241=DIRECTION('ref_axis',(-0.913545457642601,0.,-0.406736643075801));
#6242=DIRECTION('',(0.913545457642601,0.,0.406736643075801));
#6243=DIRECTION('',(0.,1.,0.));
#6244=DIRECTION('',(-0.913545457642601,0.,-0.406736643075801));
#6245=DIRECTION('',(0.,-1.,0.));
#6246=DIRECTION('center_axis',(0.,-1.,0.));
#6247=DIRECTION('ref_axis',(1.,0.,0.));
#6248=DIRECTION('center_axis',(0.,-1.,0.));
#6249=DIRECTION('ref_axis',(1.,0.,0.));
#6250=DIRECTION('',(0.,-1.,0.));
#6251=DIRECTION('center_axis',(0.,1.,0.));
#6252=DIRECTION('ref_axis',(1.,0.,0.));
#6253=DIRECTION('center_axis',(0.,-1.,0.));
#6254=DIRECTION('ref_axis',(1.,0.,0.));
#6255=DIRECTION('center_axis',(0.,1.,0.));
#6256=DIRECTION('ref_axis',(1.,0.,0.));
#6257=DIRECTION('',(0.,1.,0.));
#6258=DIRECTION('center_axis',(0.,-1.,0.));
#6259=DIRECTION('ref_axis',(1.,0.,0.));
#6260=DIRECTION('center_axis',(0.,-1.,0.));
#6261=DIRECTION('ref_axis',(1.,0.,0.));
#6262=DIRECTION('center_axis',(0.,-1.,0.));
#6263=DIRECTION('ref_axis',(1.,0.,0.));
#6264=DIRECTION('',(0.,1.,0.));
#6265=DIRECTION('center_axis',(0.,1.,0.));
#6266=DIRECTION('ref_axis',(1.,0.,0.));
#6267=DIRECTION('center_axis',(0.,-1.,0.));
#6268=DIRECTION('ref_axis',(1.,0.,0.));
#6269=DIRECTION('center_axis',(0.,1.,0.));
#6270=DIRECTION('ref_axis',(1.,0.,0.));
#6271=DIRECTION('',(0.,-1.,0.));
#6272=DIRECTION('center_axis',(0.,-1.,0.));
#6273=DIRECTION('ref_axis',(1.,0.,0.));
#6274=DIRECTION('center_axis',(0.207911690817759,0.,0.978147600733806));
#6275=DIRECTION('ref_axis',(-0.978147600733806,0.,0.207911690817759));
#6276=DIRECTION('',(0.978147600733806,0.,-0.207911690817759));
#6277=DIRECTION('',(-0.978147600733806,0.,0.207911690817759));
#6278=DIRECTION('center_axis',(-0.207911690817759,0.,-0.978147600733806));
#6279=DIRECTION('ref_axis',(0.978147600733806,0.,-0.207911690817759));
#6280=DIRECTION('',(-0.978147600733806,0.,0.207911690817759));
#6281=DIRECTION('',(0.,1.,0.));
#6282=DIRECTION('',(0.978147600733806,0.,-0.207911690817759));
#6283=DIRECTION('',(0.,-1.,0.));
#6284=DIRECTION('center_axis',(0.,-1.,0.));
#6285=DIRECTION('ref_axis',(-1.,0.,1.22464679914735E-16));
#6286=DIRECTION('center_axis',(0.,1.,0.));
#6287=DIRECTION('ref_axis',(1.,0.,0.));
#6288=DIRECTION('',(0.,1.,0.));
#6289=DIRECTION('center_axis',(0.,-1.,0.));
#6290=DIRECTION('ref_axis',(1.,0.,0.));
#6291=DIRECTION('center_axis',(0.,-1.,0.));
#6292=DIRECTION('ref_axis',(-1.,0.,5.66553889764798E-16));
#6293=DIRECTION('center_axis',(0.,1.,0.));
#6294=DIRECTION('ref_axis',(1.,0.,0.));
#6295=DIRECTION('',(0.,-1.,0.));
#6296=DIRECTION('center_axis',(0.,-1.,0.));
#6297=DIRECTION('ref_axis',(1.,0.,0.));
#6298=DIRECTION('center_axis',(0.743144825477395,0.,-0.669130606358858));
#6299=DIRECTION('ref_axis',(0.669130606358858,0.,0.743144825477395));
#6300=DIRECTION('',(-0.669130606358858,0.,-0.743144825477395));
#6301=DIRECTION('',(0.669130606358858,0.,0.743144825477395));
#6302=DIRECTION('center_axis',(-0.743144825477395,0.,0.669130606358858));
#6303=DIRECTION('ref_axis',(-0.669130606358858,0.,-0.743144825477395));
#6304=DIRECTION('',(0.669130606358858,0.,0.743144825477395));
#6305=DIRECTION('',(-0.669130606358858,0.,-0.743144825477395));
#6306=DIRECTION('center_axis',(-0.20791169081776,0.,0.978147600733806));
#6307=DIRECTION('ref_axis',(-0.978147600733805,0.,-0.20791169081776));
#6308=DIRECTION('',(0.978147600733805,0.,0.20791169081776));
#6309=DIRECTION('',(-0.978147600733805,0.,-0.20791169081776));
#6310=DIRECTION('center_axis',(0.20791169081776,0.,-0.978147600733806));
#6311=DIRECTION('ref_axis',(0.978147600733805,0.,0.20791169081776));
#6312=DIRECTION('',(-0.978147600733805,0.,-0.20791169081776));
#6313=DIRECTION('',(0.,1.,0.));
#6314=DIRECTION('',(0.978147600733805,0.,0.20791169081776));
#6315=DIRECTION('',(0.,-1.,0.));
#6316=DIRECTION('center_axis',(0.,-1.,0.));
#6317=DIRECTION('ref_axis',(1.,0.,0.));
#6318=DIRECTION('center_axis',(0.,1.,0.));
#6319=DIRECTION('ref_axis',(1.,0.,0.));
#6320=DIRECTION('',(0.,1.,0.));
#6321=DIRECTION('center_axis',(0.,-1.,0.));
#6322=DIRECTION('ref_axis',(1.,0.,0.));
#6323=DIRECTION('center_axis',(0.,-1.,0.));
#6324=DIRECTION('ref_axis',(1.,0.,0.));
#6325=DIRECTION('center_axis',(0.,1.,0.));
#6326=DIRECTION('ref_axis',(1.,0.,0.));
#6327=DIRECTION('',(0.,-1.,0.));
#6328=DIRECTION('center_axis',(0.,-1.,0.));
#6329=DIRECTION('ref_axis',(1.,0.,0.));
#6330=DIRECTION('center_axis',(0.994521895368273,0.,0.104528463267654));
#6331=DIRECTION('ref_axis',(-0.104528463267654,0.,0.994521895368273));
#6332=DIRECTION('',(0.104528463267654,0.,-0.994521895368273));
#6333=DIRECTION('',(-0.104528463267654,0.,0.994521895368273));
#6334=DIRECTION('center_axis',(-0.994521895368273,0.,-0.104528463267654));
#6335=DIRECTION('ref_axis',(0.104528463267654,0.,-0.994521895368273));
#6336=DIRECTION('',(-0.104528463267654,0.,0.994521895368273));
#6337=DIRECTION('',(0.104528463267654,0.,-0.994521895368273));
#6338=DIRECTION('center_axis',(0.99782096176235,0.,0.0659797564989427));
#6339=DIRECTION('ref_axis',(-0.0659797564989427,0.,0.99782096176235));
#6340=DIRECTION('',(0.0659797564989427,0.,-0.997820961762349));
#6341=DIRECTION('',(0.,1.,0.));
#6342=DIRECTION('',(-0.0659797564989426,0.,0.997820961762349));
#6343=DIRECTION('',(0.,-1.,0.));
#6344=DIRECTION('center_axis',(0.219561147704001,0.,-0.975598740476279));
#6345=DIRECTION('ref_axis',(0.975598740476279,0.,0.219561147704001));
#6346=DIRECTION('',(-0.975598740476279,0.,-0.219561147704001));
#6347=DIRECTION('',(0.975598740476279,0.,0.219561147704001));
#6348=DIRECTION('',(0.,-1.,0.));
#6349=DIRECTION('center_axis',(-0.925168275473212,0.,-0.379557192077721));
#6350=DIRECTION('ref_axis',(0.379557192077721,0.,-0.925168275473212));
#6351=DIRECTION('',(-0.379557192077721,0.,0.925168275473211));
#6352=DIRECTION('',(0.379557192077721,0.,-0.925168275473211));
#6353=DIRECTION('',(0.,-1.,0.));
#6354=DIRECTION('center_axis',(0.,-1.,0.));
#6355=DIRECTION('ref_axis',(1.,0.,0.));
#6356=DIRECTION('center_axis',(0.,1.,0.));
#6357=DIRECTION('ref_axis',(1.,0.,0.));
#6358=DIRECTION('',(0.,-1.,0.));
#6359=DIRECTION('center_axis',(0.,-1.,0.));
#6360=DIRECTION('ref_axis',(1.,0.,0.));
#6361=DIRECTION('center_axis',(0.,-1.,0.));
#6362=DIRECTION('ref_axis',(1.,0.,0.));
#6363=DIRECTION('center_axis',(0.,-1.,0.));
#6364=DIRECTION('ref_axis',(1.,0.,0.));
#6365=DIRECTION('',(0.,1.,0.));
#6366=DIRECTION('center_axis',(0.,1.,0.));
#6367=DIRECTION('ref_axis',(1.,0.,0.));
#6368=DIRECTION('center_axis',(0.98973414244318,0.,-0.142920702776971));
#6369=DIRECTION('ref_axis',(0.142920702776971,0.,0.98973414244318));
#6370=DIRECTION('',(-0.142920702776971,0.,-0.98973414244318));
#6371=DIRECTION('',(0.142920702776971,0.,0.98973414244318));
#6372=DIRECTION('',(0.,-1.,0.));
#6373=DIRECTION('center_axis',(0.0119248261489294,0.,-0.999928896732822));
#6374=DIRECTION('ref_axis',(0.999928896732822,0.,0.0119248261489294));
#6375=DIRECTION('',(-0.999928896732822,0.,-0.0119248261489294));
#6376=DIRECTION('',(0.999928896732822,0.,0.0119248261489294));
#6377=DIRECTION('',(0.,-1.,0.));
#6378=DIRECTION('center_axis',(-0.983865506496074,0.,-0.178909656327497));
#6379=DIRECTION('ref_axis',(0.178909656327497,0.,-0.983865506496074));
#6380=DIRECTION('',(-0.178909656327497,0.,0.983865506496074));
#6381=DIRECTION('',(0.178909656327497,0.,-0.983865506496074));
#6382=DIRECTION('',(0.,-1.,0.));
#6383=DIRECTION('center_axis',(0.,-1.,0.));
#6384=DIRECTION('ref_axis',(1.,0.,0.));
#6385=DIRECTION('center_axis',(0.,-1.,0.));
#6386=DIRECTION('ref_axis',(1.,0.,0.));
#6387=DIRECTION('',(0.,1.,0.));
#6388=DIRECTION('center_axis',(0.,1.,0.));
#6389=DIRECTION('ref_axis',(1.,0.,0.));
#6390=DIRECTION('center_axis',(0.846036043229222,0.,-0.533125701459835));
#6391=DIRECTION('ref_axis',(0.533125701459835,0.,0.846036043229222));
#6392=DIRECTION('',(-0.533125701459835,0.,-0.846036043229222));
#6393=DIRECTION('',(0.,1.,0.));
#6394=DIRECTION('',(0.533125701459835,0.,0.846036043229222));
#6395=DIRECTION('',(0.,-1.,0.));
#6396=DIRECTION('center_axis',(-0.395813852010064,0.,-0.918330765332925));
#6397=DIRECTION('ref_axis',(0.918330765332925,0.,-0.395813852010064));
#6398=DIRECTION('',(-0.918330765332925,0.,0.395813852010064));
#6399=DIRECTION('',(0.918330765332925,0.,-0.395813852010064));
#6400=DIRECTION('',(0.,-1.,0.));
#6401=DIRECTION('center_axis',(-0.971574977419217,0.,0.236732049483902));
#6402=DIRECTION('ref_axis',(-0.236732049483902,0.,-0.971574977419217));
#6403=DIRECTION('',(0.236732049483902,0.,0.971574977419217));
#6404=DIRECTION('',(-0.236732049483902,0.,-0.971574977419217));
#6405=DIRECTION('',(0.,-1.,0.));
#6406=DIRECTION('center_axis',(0.,-1.,0.));
#6407=DIRECTION('ref_axis',(1.,0.,0.));
#6408=DIRECTION('center_axis',(0.,1.,0.));
#6409=DIRECTION('ref_axis',(1.,0.,0.));
#6410=DIRECTION('',(0.,-1.,0.));
#6411=DIRECTION('center_axis',(0.,-1.,0.));
#6412=DIRECTION('ref_axis',(1.,0.,0.));
#6413=DIRECTION('center_axis',(0.,-1.,0.));
#6414=DIRECTION('ref_axis',(1.,0.,0.));
#6415=DIRECTION('center_axis',(0.,-1.,0.));
#6416=DIRECTION('ref_axis',(1.,0.,0.));
#6417=DIRECTION('',(0.,1.,0.));
#6418=DIRECTION('center_axis',(0.,1.,0.));
#6419=DIRECTION('ref_axis',(1.,0.,0.));
#6420=DIRECTION('center_axis',(0.556050626144771,0.,-0.831148423065344));
#6421=DIRECTION('ref_axis',(0.831148423065344,0.,0.556050626144771));
#6422=DIRECTION('',(-0.831148423065344,0.,-0.556050626144771));
#6423=DIRECTION('',(0.,1.,0.));
#6424=DIRECTION('',(0.831148423065344,0.,0.556050626144771));
#6425=DIRECTION('',(0.,-1.,0.));
#6426=DIRECTION('center_axis',(-0.735112719300559,0.,-0.677944901833872));
#6427=DIRECTION('ref_axis',(0.677944901833872,0.,-0.735112719300559));
#6428=DIRECTION('',(-0.677944901833872,0.,0.735112719300559));
#6429=DIRECTION('',(0.677944901833871,0.,-0.735112719300559));
#6430=DIRECTION('',(0.,-1.,0.));
#6431=DIRECTION('center_axis',(-0.791290308265002,0.,0.61144063329638));
#6432=DIRECTION('ref_axis',(-0.61144063329638,0.,-0.791290308265002));
#6433=DIRECTION('',(0.61144063329638,0.,0.791290308265002));
#6434=DIRECTION('',(-0.61144063329638,0.,-0.791290308265002));
#6435=DIRECTION('',(0.,-1.,0.));
#6436=DIRECTION('center_axis',(0.,-1.,0.));
#6437=DIRECTION('ref_axis',(1.,0.,0.));
#6438=DIRECTION('center_axis',(0.,1.,0.));
#6439=DIRECTION('ref_axis',(1.,0.,0.));
#6440=DIRECTION('',(0.,-1.,0.));
#6441=DIRECTION('center_axis',(0.,-1.,0.));
#6442=DIRECTION('ref_axis',(1.,0.,0.));
#6443=DIRECTION('center_axis',(0.,-1.,0.));
#6444=DIRECTION('ref_axis',(1.,0.,0.));
#6445=DIRECTION('center_axis',(0.,-1.,0.));
#6446=DIRECTION('ref_axis',(1.,0.,0.));
#6447=DIRECTION('',(0.,1.,0.));
#6448=DIRECTION('center_axis',(0.,1.,0.));
#6449=DIRECTION('ref_axis',(1.,0.,0.));
#6450=DIRECTION('center_axis',(0.716705059810068,0.,-0.69737641001302));
#6451=DIRECTION('ref_axis',(0.69737641001302,0.,0.716705059810068));
#6452=DIRECTION('',(-0.69737641001302,0.,-0.716705059810068));
#6453=DIRECTION('',(0.69737641001302,0.,0.716705059810068));
#6454=DIRECTION('',(0.,-1.,0.));
#6455=DIRECTION('center_axis',(-0.578096071831185,0.,-0.815968707569937));
#6456=DIRECTION('ref_axis',(0.815968707569937,0.,-0.578096071831185));
#6457=DIRECTION('',(-0.815968707569937,0.,0.578096071831185));
#6458=DIRECTION('',(0.815968707569937,0.,-0.578096071831185));
#6459=DIRECTION('',(0.,-1.,0.));
#6460=DIRECTION('center_axis',(-0.901124372416657,0.,0.433560682530931));
#6461=DIRECTION('ref_axis',(-0.433560682530931,0.,-0.901124372416657));
#6462=DIRECTION('',(0.433560682530931,0.,0.901124372416657));
#6463=DIRECTION('',(-0.433560682530931,0.,-0.901124372416657));
#6464=DIRECTION('center_axis',(0.962298216976301,0.,0.271996583809855));
#6465=DIRECTION('ref_axis',(-0.271996583809855,0.,0.962298216976301));
#6466=DIRECTION('',(0.271996583809855,0.,-0.962298216976301));
#6467=DIRECTION('',(-0.271996583809855,0.,0.962298216976301));
#6468=DIRECTION('',(0.,-1.,0.));
#6469=DIRECTION('center_axis',(0.417601593533129,0.,-0.908630237818768));
#6470=DIRECTION('ref_axis',(0.908630237818768,0.,0.417601593533129));
#6471=DIRECTION('',(-0.908630237818768,0.,-0.417601593533129));
#6472=DIRECTION('',(0.908630237818768,0.,0.417601593533129));
#6473=DIRECTION('',(0.,-1.,0.));
#6474=DIRECTION('center_axis',(-0.826036751362234,0.,-0.563616257216669));
#6475=DIRECTION('ref_axis',(0.563616257216669,0.,-0.826036751362234));
#6476=DIRECTION('',(-0.563616257216669,0.,0.826036751362234));
#6477=DIRECTION('',(0.563616257216669,0.,-0.826036751362234));
#6478=DIRECTION('center_axis',(0.938391191827905,0.,-0.34557484153191));
#6479=DIRECTION('ref_axis',(0.34557484153191,0.,0.938391191827905));
#6480=DIRECTION('',(-0.34557484153191,0.,-0.938391191827905));
#6481=DIRECTION('',(0.34557484153191,0.,0.938391191827905));
#6482=DIRECTION('',(0.,-1.,0.));
#6483=DIRECTION('center_axis',(-0.196232667530514,0.,-0.980557362010943));
#6484=DIRECTION('ref_axis',(0.980557362010943,0.,-0.196232667530514));
#6485=DIRECTION('',(-0.980557362010943,0.,0.196232667530514));
#6486=DIRECTION('',(0.980557362010943,0.,-0.196232667530514));
#6487=DIRECTION('',(0.,-1.,0.));
#6488=DIRECTION('center_axis',(-0.99956309377456,0.,0.0295570899080193));
#6489=DIRECTION('ref_axis',(-0.0295570899080193,0.,-0.99956309377456));
#6490=DIRECTION('',(0.0295570899080193,0.,0.99956309377456));
#6491=DIRECTION('',(-0.0295570899080193,0.,-0.99956309377456));
#6492=DIRECTION('center_axis',(0.371094111890008,0.,-0.928595261737086));
#6493=DIRECTION('ref_axis',(0.928595261737086,0.,0.371094111890008));
#6494=DIRECTION('',(-0.928595261737086,0.,-0.371094111890008));
#6495=DIRECTION('',(0.928595261737086,0.,0.371094111890008));
#6496=DIRECTION('',(0.,-1.,0.));
#6497=DIRECTION('center_axis',(-0.860001413474305,0.,-0.510291650747097));
#6498=DIRECTION('ref_axis',(0.510291650747097,0.,-0.860001413474305));
#6499=DIRECTION('',(-0.510291650747097,0.,0.860001413474305));
#6500=DIRECTION('',(0.510291650747097,0.,-0.860001413474305));
#6501=DIRECTION('',(0.,-1.,0.));
#6502=DIRECTION('center_axis',(-0.646873060609993,0.,0.762597694369096));
#6503=DIRECTION('ref_axis',(-0.762597694369096,0.,-0.646873060609993));
#6504=DIRECTION('',(0.762597694369096,0.,0.646873060609993));
#6505=DIRECTION('',(-0.762597694369096,0.,-0.646873060609993));
#6506=DIRECTION('',(0.,-1.,0.));
#6507=DIRECTION('center_axis',(0.,-1.,0.));
#6508=DIRECTION('ref_axis',(1.,0.,0.));
#6509=DIRECTION('center_axis',(0.,-1.,0.));
#6510=DIRECTION('ref_axis',(1.,0.,0.));
#6511=DIRECTION('',(0.,1.,0.));
#6512=DIRECTION('center_axis',(0.,1.,0.));
#6513=DIRECTION('ref_axis',(1.,0.,0.));
#6514=DIRECTION('center_axis',(-0.587785252292473,0.,0.809016994374947));
#6515=DIRECTION('ref_axis',(-0.809016994374947,0.,-0.587785252292473));
#6516=DIRECTION('',(0.809016994374947,0.,0.587785252292473));
#6517=DIRECTION('',(-0.809016994374947,0.,-0.587785252292473));
#6518=DIRECTION('center_axis',(0.587785252292473,0.,-0.809016994374947));
#6519=DIRECTION('ref_axis',(0.809016994374947,0.,0.587785252292473));
#6520=DIRECTION('',(-0.809016994374947,0.,-0.587785252292473));
#6521=DIRECTION('',(0.,1.,0.));
#6522=DIRECTION('',(0.809016994374947,0.,0.587785252292473));
#6523=DIRECTION('',(0.,-1.,0.));
#6524=DIRECTION('center_axis',(0.,-1.,0.));
#6525=DIRECTION('ref_axis',(1.,0.,0.));
#6526=DIRECTION('center_axis',(0.,1.,0.));
#6527=DIRECTION('ref_axis',(1.,0.,0.));
#6528=DIRECTION('',(0.,1.,0.));
#6529=DIRECTION('center_axis',(0.,-1.,0.));
#6530=DIRECTION('ref_axis',(1.,0.,0.));
#6531=DIRECTION('center_axis',(0.,-1.,0.));
#6532=DIRECTION('ref_axis',(1.,0.,0.));
#6533=DIRECTION('center_axis',(0.,1.,0.));
#6534=DIRECTION('ref_axis',(1.,0.,0.));
#6535=DIRECTION('',(0.,-1.,0.));
#6536=DIRECTION('center_axis',(0.,-1.,0.));
#6537=DIRECTION('ref_axis',(1.,0.,0.));
#6538=DIRECTION('center_axis',(-0.994521895368273,0.,0.104528463267653));
#6539=DIRECTION('ref_axis',(-0.104528463267653,0.,-0.994521895368273));
#6540=DIRECTION('',(0.104528463267653,0.,0.994521895368273));
#6541=DIRECTION('',(0.,1.,0.));
#6542=DIRECTION('',(-0.104528463267653,0.,-0.994521895368273));
#6543=DIRECTION('',(0.,-1.,0.));
#6544=DIRECTION('center_axis',(0.994521895368273,0.,-0.104528463267653));
#6545=DIRECTION('ref_axis',(0.104528463267653,0.,0.994521895368273));
#6546=DIRECTION('',(-0.104528463267653,0.,-0.994521895368273));
#6547=DIRECTION('',(0.104528463267653,0.,0.994521895368273));
#6548=DIRECTION('center_axis',(0.,-1.,0.));
#6549=DIRECTION('ref_axis',(1.,0.,0.));
#6550=DIRECTION('center_axis',(0.,-1.,0.));
#6551=DIRECTION('ref_axis',(1.,0.,0.));
#6552=DIRECTION('',(0.,-1.,0.));
#6553=DIRECTION('center_axis',(0.,1.,0.));
#6554=DIRECTION('ref_axis',(1.,0.,0.));
#6555=DIRECTION('center_axis',(0.,-1.,0.));
#6556=DIRECTION('ref_axis',(1.,0.,0.));
#6557=DIRECTION('center_axis',(0.,-1.,0.));
#6558=DIRECTION('ref_axis',(1.,0.,0.));
#6559=DIRECTION('',(0.,1.,0.));
#6560=DIRECTION('center_axis',(0.,1.,0.));
#6561=DIRECTION('ref_axis',(1.,0.,0.));
#6562=DIRECTION('center_axis',(-0.866025403784439,0.,0.5));
#6563=DIRECTION('ref_axis',(-0.5,0.,-0.866025403784439));
#6564=DIRECTION('',(0.5,0.,0.866025403784439));
#6565=DIRECTION('',(-0.5,0.,-0.866025403784439));
#6566=DIRECTION('center_axis',(0.866025403784439,0.,-0.5));
#6567=DIRECTION('ref_axis',(0.5,0.,0.866025403784439));
#6568=DIRECTION('',(-0.5,0.,-0.866025403784439));
#6569=DIRECTION('',(0.5,0.,0.866025403784439));
#6570=DIRECTION('center_axis',(-0.245593157166233,0.,-0.969372993822874));
#6571=DIRECTION('ref_axis',(0.969372993822874,0.,-0.245593157166233));
#6572=DIRECTION('',(-0.969372993822874,0.,0.245593157166233));
#6573=DIRECTION('',(0.,1.,0.));
#6574=DIRECTION('',(0.969372993822874,0.,-0.245593157166233));
#6575=DIRECTION('',(0.,-1.,0.));
#6576=DIRECTION('center_axis',(-0.995697665364314,0.,0.0926615302488315));
#6577=DIRECTION('ref_axis',(-0.0926615302488315,0.,-0.995697665364314));
#6578=DIRECTION('',(0.0926615302488314,0.,0.995697665364314));
#6579=DIRECTION('',(-0.0926615302488314,0.,-0.995697665364314));
#6580=DIRECTION('',(0.,-1.,0.));
#6581=DIRECTION('center_axis',(-0.0750876210544224,0.,0.997176939747599));
#6582=DIRECTION('ref_axis',(-0.997176939747599,0.,-0.0750876210544224));
#6583=DIRECTION('',(0.997176939747599,0.,0.0750876210544224));
#6584=DIRECTION('',(-0.997176939747599,0.,-0.0750876210544224));
#6585=DIRECTION('',(0.,-1.,0.));
#6586=DIRECTION('center_axis',(0.,-1.,0.));
#6587=DIRECTION('ref_axis',(1.,0.,0.));
#6588=DIRECTION('center_axis',(0.,1.,0.));
#6589=DIRECTION('ref_axis',(1.,0.,0.));
#6590=DIRECTION('',(0.,-1.,0.));
#6591=DIRECTION('center_axis',(0.,-1.,0.));
#6592=DIRECTION('ref_axis',(1.,0.,0.));
#6593=DIRECTION('center_axis',(0.,-1.,0.));
#6594=DIRECTION('ref_axis',(1.,0.,0.));
#6595=DIRECTION('center_axis',(0.,-1.,0.));
#6596=DIRECTION('ref_axis',(1.,0.,0.));
#6597=DIRECTION('',(0.,1.,0.));
#6598=DIRECTION('center_axis',(0.,1.,0.));
#6599=DIRECTION('ref_axis',(1.,0.,0.));
#6600=DIRECTION('center_axis',(-0.441770335617579,0.,-0.897128179564287));
#6601=DIRECTION('ref_axis',(0.897128179564287,0.,-0.441770335617579));
#6602=DIRECTION('',(-0.897128179564287,0.,0.441770335617579));
#6603=DIRECTION('',(0.897128179564287,0.,-0.441770335617579));
#6604=DIRECTION('',(0.,-1.,0.));
#6605=DIRECTION('center_axis',(-0.95467386700456,0.,0.297653838642407));
#6606=DIRECTION('ref_axis',(-0.297653838642407,0.,-0.95467386700456));
#6607=DIRECTION('',(0.297653838642407,0.,0.95467386700456));
#6608=DIRECTION('',(-0.297653838642407,0.,-0.95467386700456));
#6609=DIRECTION('',(0.,-1.,0.));
#6610=DIRECTION('center_axis',(0.13387796720821,0.,0.990997825374101));
#6611=DIRECTION('ref_axis',(-0.990997825374101,0.,0.13387796720821));
#6612=DIRECTION('',(0.990997825374101,0.,-0.13387796720821));
#6613=DIRECTION('',(-0.990997825374101,0.,0.13387796720821));
#6614=DIRECTION('',(0.,-1.,0.));
#6615=DIRECTION('center_axis',(0.,-1.,0.));
#6616=DIRECTION('ref_axis',(1.,0.,0.));
#6617=DIRECTION('center_axis',(0.,-1.,0.));
#6618=DIRECTION('ref_axis',(1.,0.,0.));
#6619=DIRECTION('',(0.,1.,0.));
#6620=DIRECTION('center_axis',(0.,1.,0.));
#6621=DIRECTION('ref_axis',(1.,0.,0.));
#6622=DIRECTION('center_axis',(-0.884718422489227,0.,-0.466125855223859));
#6623=DIRECTION('ref_axis',(0.466125855223859,0.,-0.884718422489227));
#6624=DIRECTION('',(-0.466125855223859,0.,0.884718422489227));
#6625=DIRECTION('',(0.,1.,0.));
#6626=DIRECTION('',(0.466125855223859,0.,-0.884718422489227));
#6627=DIRECTION('',(0.,-1.,0.));
#6628=DIRECTION('center_axis',(-0.597390845850087,0.,0.801950233676952));
#6629=DIRECTION('ref_axis',(-0.801950233676952,0.,-0.597390845850087));
#6630=DIRECTION('',(0.801950233676952,0.,0.597390845850087));
#6631=DIRECTION('',(-0.801950233676952,0.,-0.597390845850087));
#6632=DIRECTION('',(0.,-1.,0.));
#6633=DIRECTION('center_axis',(0.690803457452622,0.,0.723042587384383));
#6634=DIRECTION('ref_axis',(-0.723042587384383,0.,0.690803457452622));
#6635=DIRECTION('',(0.723042587384383,0.,-0.690803457452622));
#6636=DIRECTION('',(-0.723042587384383,0.,0.690803457452622));
#6637=DIRECTION('',(0.,-1.,0.));
#6638=DIRECTION('center_axis',(0.,-1.,0.));
#6639=DIRECTION('ref_axis',(1.,0.,0.));
#6640=DIRECTION('center_axis',(0.,1.,0.));
#6641=DIRECTION('ref_axis',(1.,0.,0.));
#6642=DIRECTION('',(0.,-1.,0.));
#6643=DIRECTION('center_axis',(0.,-1.,0.));
#6644=DIRECTION('ref_axis',(1.,0.,0.));
#6645=DIRECTION('center_axis',(0.,-1.,0.));
#6646=DIRECTION('ref_axis',(1.,0.,0.));
#6647=DIRECTION('center_axis',(0.,-1.,0.));
#6648=DIRECTION('ref_axis',(1.,0.,0.));
#6649=DIRECTION('',(0.,1.,0.));
#6650=DIRECTION('center_axis',(0.,1.,0.));
#6651=DIRECTION('ref_axis',(1.,0.,0.));
#6652=DIRECTION('center_axis',(-0.618640030553172,0.,-0.785674558960115));
#6653=DIRECTION('ref_axis',(0.785674558960115,0.,-0.618640030553172));
#6654=DIRECTION('',(-0.785674558960115,0.,0.618640030553172));
#6655=DIRECTION('',(0.785674558960114,0.,-0.618640030553172));
#6656=DIRECTION('',(0.,-1.,0.));
#6657=DIRECTION('center_axis',(-0.871926239623235,0.,0.489637245985725));
#6658=DIRECTION('ref_axis',(-0.489637245985725,0.,-0.871926239623235));
#6659=DIRECTION('',(0.489637245985725,0.,0.871926239623235));
#6660=DIRECTION('',(-0.489637245985725,0.,-0.871926239623235));
#6661=DIRECTION('',(0.,-1.,0.));
#6662=DIRECTION('center_axis',(0.336992445886081,0.,0.941507350696593));
#6663=DIRECTION('ref_axis',(-0.941507350696593,0.,0.336992445886081));
#6664=DIRECTION('',(0.941507350696593,0.,-0.336992445886081));
#6665=DIRECTION('',(-0.941507350696593,0.,0.336992445886081));
#6666=DIRECTION('',(0.,-1.,0.));
#6667=DIRECTION('center_axis',(0.,-1.,0.));
#6668=DIRECTION('ref_axis',(1.,0.,0.));
#6669=DIRECTION('center_axis',(0.,-1.,0.));
#6670=DIRECTION('ref_axis',(1.,0.,0.));
#6671=DIRECTION('',(0.,1.,0.));
#6672=DIRECTION('center_axis',(0.,1.,0.));
#6673=DIRECTION('ref_axis',(1.,0.,0.));
#6674=DIRECTION('center_axis',(0.169919004238536,0.,-0.985458031576477));
#6675=DIRECTION('ref_axis',(0.985458031576477,0.,0.169919004238536));
#6676=DIRECTION('',(-0.985458031576477,0.,-0.169919004238536));
#6677=DIRECTION('',(0.985458031576477,0.,0.169919004238536));
#6678=DIRECTION('',(0.,-1.,0.));
#6679=DIRECTION('center_axis',(-0.947303919134588,0.,-0.32033620587166));
#6680=DIRECTION('ref_axis',(0.32033620587166,0.,-0.947303919134588));
#6681=DIRECTION('',(-0.32033620587166,0.,0.947303919134588));
#6682=DIRECTION('',(0.32033620587166,0.,-0.947303919134588));
#6683=DIRECTION('',(0.,-1.,0.));
#6684=DIRECTION('center_axis',(-0.474184356164995,0.,0.880425576848145));
#6685=DIRECTION('ref_axis',(-0.880425576848145,0.,-0.474184356164995));
#6686=DIRECTION('',(0.880425576848145,0.,0.474184356164995));
#6687=DIRECTION('',(-0.880425576848145,0.,-0.474184356164995));
#6688=DIRECTION('',(0.,-1.,0.));
#6689=DIRECTION('center_axis',(0.,-1.,0.));
#6690=DIRECTION('ref_axis',(1.,0.,0.));
#6691=DIRECTION('center_axis',(0.,-1.,0.));
#6692=DIRECTION('ref_axis',(1.,0.,0.));
#6693=DIRECTION('',(0.,1.,0.));
#6694=DIRECTION('center_axis',(0.,1.,0.));
#6695=DIRECTION('ref_axis',(1.,0.,0.));
#6696=DIRECTION('center_axis',(-0.962298216976301,0.,-0.271996583809855));
#6697=DIRECTION('ref_axis',(0.271996583809855,0.,-0.962298216976301));
#6698=DIRECTION('',(-0.271996583809855,0.,0.962298216976301));
#6699=DIRECTION('',(0.271996583809855,0.,-0.962298216976301));
#6700=DIRECTION('',(0.,-1.,0.));
#6701=DIRECTION('center_axis',(-0.417601593533129,0.,0.908630237818768));
#6702=DIRECTION('ref_axis',(-0.908630237818768,0.,-0.417601593533129));
#6703=DIRECTION('',(0.908630237818768,0.,0.417601593533129));
#6704=DIRECTION('',(-0.908630237818768,0.,-0.417601593533129));
#6705=DIRECTION('',(0.,-1.,0.));
#6706=DIRECTION('center_axis',(0.826036751362234,0.,0.563616257216669));
#6707=DIRECTION('ref_axis',(-0.563616257216669,0.,0.826036751362234));
#6708=DIRECTION('',(0.563616257216669,0.,-0.826036751362234));
#6709=DIRECTION('',(-0.563616257216669,0.,0.826036751362234));
#6710=DIRECTION('center_axis',(-0.768472187589368,0.,-0.639883190044567));
#6711=DIRECTION('ref_axis',(0.639883190044567,0.,-0.768472187589368));
#6712=DIRECTION('',(-0.639883190044567,0.,0.768472187589368));
#6713=DIRECTION('',(0.639883190044567,0.,-0.768472187589368));
#6714=DIRECTION('',(0.,-1.,0.));
#6715=DIRECTION('center_axis',(-0.751071251604073,0.,0.660221156139283));
#6716=DIRECTION('ref_axis',(-0.660221156139283,0.,-0.751071251604073));
#6717=DIRECTION('',(0.660221156139282,0.,0.751071251604074));
#6718=DIRECTION('',(-0.660221156139282,0.,-0.751071251604074));
#6719=DIRECTION('',(0.,-1.,0.));
#6720=DIRECTION('center_axis',(0.525378737609565,0.,0.850868486940126));
#6721=DIRECTION('ref_axis',(-0.850868486940126,0.,0.525378737609565));
#6722=DIRECTION('',(0.850868486940126,0.,-0.525378737609565));
#6723=DIRECTION('',(-0.850868486940126,0.,0.525378737609565));
#6724=DIRECTION('center_axis',(-0.0386823792600045,0.,-0.999251556683694));
#6725=DIRECTION('ref_axis',(0.999251556683694,0.,-0.0386823792600045));
#6726=DIRECTION('',(-0.999251556683694,0.,0.0386823792600045));
#6727=DIRECTION('',(0.999251556683694,0.,-0.0386823792600045));
#6728=DIRECTION('',(0.,-1.,0.));
#6729=DIRECTION('center_axis',(-0.993204697860151,0.,-0.116380531655973));
#6730=DIRECTION('ref_axis',(0.116380531655973,0.,-0.993204697860151));
#6731=DIRECTION('',(-0.116380531655973,0.,0.993204697860151));
#6732=DIRECTION('',(0.116380531655973,0.,-0.993204697860151));
#6733=DIRECTION('',(0.,-1.,0.));
#6734=DIRECTION('center_axis',(-0.280771519966595,0.,0.959774636868285));
#6735=DIRECTION('ref_axis',(-0.959774636868285,0.,-0.280771519966595));
#6736=DIRECTION('',(0.959774636868285,0.,0.280771519966595));
#6737=DIRECTION('',(-0.959774636868285,0.,-0.280771519966595));
#6738=DIRECTION('center_axis',(0.,0.,-1.));
#6739=DIRECTION('ref_axis',(1.,0.,0.));
#6740=DIRECTION('',(-1.,0.,0.));
#6741=DIRECTION('',(1.,0.,0.));
#6742=DIRECTION('center_axis',(0.,0.,1.));
#6743=DIRECTION('ref_axis',(-1.,0.,0.));
#6744=DIRECTION('',(1.,0.,0.));
#6745=DIRECTION('',(-1.,0.,0.));
#6746=DIRECTION('center_axis',(0.,-1.,0.));
#6747=DIRECTION('ref_axis',(1.,0.,0.));
#6748=DIRECTION('center_axis',(0.,-1.,0.));
#6749=DIRECTION('ref_axis',(1.,0.,0.));
#6750=DIRECTION('',(0.,-1.,0.));
#6751=DIRECTION('center_axis',(0.,1.,0.));
#6752=DIRECTION('ref_axis',(1.,0.,0.));
#6753=DIRECTION('center_axis',(0.,1.,0.));
#6754=DIRECTION('ref_axis',(1.,0.,0.));
#6755=DIRECTION('center_axis',(0.,1.,0.));
#6756=DIRECTION('ref_axis',(1.,0.,0.));
#7248=CARTESIAN_POINT('',(0.,0.,0.));
#7249=CARTESIAN_POINT('Origin',(31.2735217236592,-4.5,50.3382969385033));
#7250=CARTESIAN_POINT('',(31.2735217236592,-2.5,50.3382969385033));
#7251=CARTESIAN_POINT('',(25.2794356395192,-2.5,49.3047581107688));
#7252=CARTESIAN_POINT('',(15.94574796428,-2.5,47.6953837235988));
#7253=CARTESIAN_POINT('',(25.2794356395192,-6.5,49.3047581107688));
#7254=CARTESIAN_POINT('',(25.2794356395192,-4.5,49.3047581107688));
#7255=CARTESIAN_POINT('',(31.2735217236592,-6.5,50.3382969385033));
#7256=CARTESIAN_POINT('',(31.5856264400152,-6.5,50.3921120386111));
#7257=CARTESIAN_POINT('',(31.2735217236592,-4.5,50.3382969385033));
#7258=CARTESIAN_POINT('Origin',(31.3062123347366,-4.5,50.2416236826399));
#7259=CARTESIAN_POINT('',(31.3062123347366,-2.5,50.2416236826399));
#7260=CARTESIAN_POINT('',(29.943512708519,-2.5,54.2714232271732));
#7261=CARTESIAN_POINT('',(31.3062123347366,-6.5,50.2416236826399));
#7262=CARTESIAN_POINT('',(31.0437587864934,-6.5,51.0177559782855));
#7263=CARTESIAN_POINT('',(31.3062123347366,-4.5,50.2416236826399));
#7264=CARTESIAN_POINT('Origin',(25.2333571880834,-4.5,46.9708726009778));
#7265=CARTESIAN_POINT('',(25.2333571880834,-2.5,46.9708726009778));
#7266=CARTESIAN_POINT('',(15.8012266428482,-2.5,41.8908648553283));
#7267=CARTESIAN_POINT('',(25.2333571880834,-6.5,46.9708726009778));
#7268=CARTESIAN_POINT('',(31.5856264400152,-6.5,50.3921120386111));
#7269=CARTESIAN_POINT('',(25.2333571880834,-4.5,46.9708726009778));
#7270=CARTESIAN_POINT('Origin',(0.,-4.5,48.6364583401654));
#7271=CARTESIAN_POINT('',(25.0282425392193,-2.5,52.2535796035455));
#7272=CARTESIAN_POINT('Origin',(0.,-2.5,48.6364583401654));
#7273=CARTESIAN_POINT('',(25.0282425392193,-6.5,52.2535796035455));
#7274=CARTESIAN_POINT('',(25.0282425392193,-4.5,52.2535796035455));
#7275=CARTESIAN_POINT('Origin',(0.,-6.5,48.6364583401654));
#7276=CARTESIAN_POINT('Origin',(0.,-4.5,48.6364583401654));
#7277=CARTESIAN_POINT('',(24.8659666539797,-6.5,44.0342639506209));
#7278=CARTESIAN_POINT('Origin',(0.,-6.5,48.6364583401654));
#7279=CARTESIAN_POINT('',(24.8659666539797,-2.5,44.0342639506209));
#7280=CARTESIAN_POINT('',(24.8659666539797,-4.5,44.0342639506209));
#7281=CARTESIAN_POINT('Origin',(0.,-2.5,48.6364583401654));
#7282=CARTESIAN_POINT('Origin',(26.3011261782795,-4.5,31.6311598314889));
#7283=CARTESIAN_POINT('',(26.3011261782795,-2.5,31.6311598314889));
#7284=CARTESIAN_POINT('',(20.8443097898499,-2.5,34.3182447567343));
#7285=CARTESIAN_POINT('',(12.3472313101976,-2.5,38.5024374922116));
#7286=CARTESIAN_POINT('',(20.8443097898499,-6.5,34.3182447567343));
#7287=CARTESIAN_POINT('',(20.8443097898499,-4.5,34.3182447567343));
#7288=CARTESIAN_POINT('',(26.3011261782795,-6.5,31.6311598314889));
#7289=CARTESIAN_POINT('',(26.5852559200301,-6.5,31.4912466125851));
#7290=CARTESIAN_POINT('',(26.3011261782795,-4.5,31.6311598314889));
#7291=CARTESIAN_POINT('Origin',(26.27075032411,-4.5,31.533734465514));
#7292=CARTESIAN_POINT('',(26.27075032411,-2.5,31.533734465514));
#7293=CARTESIAN_POINT('',(27.5369599102432,-2.5,35.5948855245611));
#7294=CARTESIAN_POINT('',(26.27075032411,-6.5,31.533734465514));
#7295=CARTESIAN_POINT('',(26.5146200605556,-6.5,32.3159050076438));
#7296=CARTESIAN_POINT('',(26.27075032411,-4.5,31.533734465514));
#7297=CARTESIAN_POINT('Origin',(19.4352080563696,-4.5,32.4571759505904));
#7298=CARTESIAN_POINT('',(19.4352080563695,-2.5,32.4571759505904));
#7299=CARTESIAN_POINT('',(8.81850051768697,-2.5,33.8914305849902));
#7300=CARTESIAN_POINT('',(19.4352080563696,-6.5,32.4571759505904));
#7301=CARTESIAN_POINT('',(26.5852559200301,-6.5,31.4912466125851));
#7302=CARTESIAN_POINT('',(19.4352080563695,-4.5,32.4571759505904));
#7303=CARTESIAN_POINT('Origin',(0.,-4.5,48.6364583401654));
#7304=CARTESIAN_POINT('',(22.3743640879347,-2.5,36.8515390576026));
#7305=CARTESIAN_POINT('Origin',(0.,-2.5,48.6364583401654));
#7306=CARTESIAN_POINT('',(22.3743640879347,-6.5,36.8515390576026));
#7307=CARTESIAN_POINT('',(22.3743640879347,-4.5,36.8515390576026));
#7308=CARTESIAN_POINT('Origin',(0.,-6.5,48.6364583401654));
#7309=CARTESIAN_POINT('Origin',(0.,-4.5,48.6364583401654));
#7310=CARTESIAN_POINT('',(17.4118876142729,-6.5,30.2973563844012));
#7311=CARTESIAN_POINT('Origin',(0.,-6.5,48.6364583401654));
#7312=CARTESIAN_POINT('',(17.4118876142729,-2.5,30.2973563844012));
#7313=CARTESIAN_POINT('',(17.4118876142729,-4.5,30.2973563844012));
#7314=CARTESIAN_POINT('Origin',(0.,-2.5,48.6364583401654));
#7315=CARTESIAN_POINT('Origin',(30.9439523809731,-4.5,43.7989769025739));
#7316=CARTESIAN_POINT('',(30.9439523809731,-2.5,43.7989769025739));
#7317=CARTESIAN_POINT('',(15.4016346984504,-2.5,44.400641041252));
#7318=CARTESIAN_POINT('',(30.9439523809731,-6.5,43.7989769025739));
#7319=CARTESIAN_POINT('',(31.2604256489094,-6.5,43.7867257943379));
#7320=CARTESIAN_POINT('',(30.9439523809731,-4.5,43.7989769025739));
#7321=CARTESIAN_POINT('Origin',(30.9558291236816,-4.5,43.697619429073));
#7322=CARTESIAN_POINT('',(30.9558291236816,-2.5,43.697619429073));
#7323=CARTESIAN_POINT('',(30.4607501907366,-2.5,47.9226793683601));
#7324=CARTESIAN_POINT('',(30.9558291236816,-6.5,43.697619429073));
#7325=CARTESIAN_POINT('',(30.8604777930494,-6.5,44.5113585328872));
#7326=CARTESIAN_POINT('',(30.9558291236816,-4.5,43.697619429073));
#7327=CARTESIAN_POINT('Origin',(24.3356530447464,-4.5,41.7609596875797));
#7328=CARTESIAN_POINT('',(24.3356530447464,-2.5,41.7609596875797));
#7329=CARTESIAN_POINT('',(14.0534441823513,-2.5,38.7530125091372));
#7330=CARTESIAN_POINT('',(24.3356530447464,-6.5,41.7609596875797));
#7331=CARTESIAN_POINT('',(31.2604256489094,-6.5,43.7867257943379));
#7332=CARTESIAN_POINT('',(24.3356530447464,-4.5,41.7609596875797));
#7333=CARTESIAN_POINT('Origin',(0.,-4.5,48.6364583401654));
#7334=CARTESIAN_POINT('',(23.3657356055148,-6.5,38.9649077690749));
#7335=CARTESIAN_POINT('Origin',(0.,-6.5,48.6364583401654));
#7336=CARTESIAN_POINT('',(23.3657356055148,-2.5,38.9649077690749));
#7337=CARTESIAN_POINT('',(23.3657356055148,-4.5,38.9649077690749));
#7338=CARTESIAN_POINT('Origin',(0.,-2.5,48.6364583401654));
#7339=CARTESIAN_POINT('Origin',(11.2825943751967,-4.5,19.419468765951));
#7340=CARTESIAN_POINT('',(11.2825943751967,-2.5,19.419468765951));
#7341=CARTESIAN_POINT('',(8.44736607249008,-2.5,24.80080233339));
#7342=CARTESIAN_POINT('',(4.03249196257661,-2.5,33.1803427820428));
#7343=CARTESIAN_POINT('',(8.44736607249008,-6.5,24.80080233339));
#7344=CARTESIAN_POINT('',(8.44736607249008,-4.5,24.80080233339));
#7345=CARTESIAN_POINT('',(11.2825943751967,-6.5,19.419468765951));
#7346=CARTESIAN_POINT('',(11.4302212382079,-6.5,19.1392693221814));
#7347=CARTESIAN_POINT('',(11.2825943751967,-4.5,19.419468765951));
#7348=CARTESIAN_POINT('Origin',(11.2007545996357,-4.5,19.3585044683007));
#7349=CARTESIAN_POINT('',(11.2007545996357,-2.5,19.3585044683007));
#7350=CARTESIAN_POINT('',(14.6122243730978,-2.5,21.8997853707532));
#7351=CARTESIAN_POINT('',(11.2007545996357,-6.5,19.3585044683007));
#7352=CARTESIAN_POINT('',(11.8577976702754,-6.5,19.84795069482));
#7353=CARTESIAN_POINT('',(11.2007545996357,-4.5,19.3585044683007));
#7354=CARTESIAN_POINT('Origin',(6.21347002554836,-4.5,24.123415259438));
#7355=CARTESIAN_POINT('',(6.21347002554835,-2.5,24.123415259438));
#7356=CARTESIAN_POINT('',(-1.53259307542216,-2.5,31.5240957520684));
#7357=CARTESIAN_POINT('',(6.21347002554835,-6.5,24.123415259438));
#7358=CARTESIAN_POINT('',(11.4302212382079,-6.5,19.1392693221814));
#7359=CARTESIAN_POINT('',(6.21347002554835,-4.5,24.123415259438));
#7360=CARTESIAN_POINT('Origin',(0.,-4.5,48.6364583401654));
#7361=CARTESIAN_POINT('',(11.1742390317241,-2.5,25.9509371229247));
#7362=CARTESIAN_POINT('Origin',(0.,-2.5,48.6364583401654));
#7363=CARTESIAN_POINT('',(11.1742390317241,-6.5,25.9509371229247));
#7364=CARTESIAN_POINT('',(11.1742390317241,-4.5,25.9509371229247));
#7365=CARTESIAN_POINT('Origin',(0.,-6.5,48.6364583401654));
#7366=CARTESIAN_POINT('Origin',(0.,-4.5,48.6364583401654));
#7367=CARTESIAN_POINT('',(3.30705931420718,-6.5,23.5653624421338));
#7368=CARTESIAN_POINT('Origin',(0.,-6.5,48.6364583401654));
#7369=CARTESIAN_POINT('',(3.30705931420717,-2.5,23.5653624421338));
#7370=CARTESIAN_POINT('',(3.30705931420717,-4.5,23.5653624421338));
#7371=CARTESIAN_POINT('Origin',(0.,-2.5,48.6364583401654));
#7372=CARTESIAN_POINT('Origin',(29.2619838336808,-4.5,37.4710780182786));
#7373=CARTESIAN_POINT('',(29.2619838336808,-2.5,37.4710780182786));
#7374=CARTESIAN_POINT('',(14.1843960910556,-2.5,41.2910239005742));
#7375=CARTESIAN_POINT('',(29.2619838336808,-6.5,37.4710780182786));
#7376=CARTESIAN_POINT('',(29.5689942527814,-6.5,37.3932961339159));
#7377=CARTESIAN_POINT('',(29.2619838336808,-4.5,37.4710780182786));
#7378=CARTESIAN_POINT('Origin',(29.2525276373731,-4.5,37.3694661350993));
#7379=CARTESIAN_POINT('',(29.2525276373731,-2.5,37.3694661350993));
#7380=CARTESIAN_POINT('',(29.6467067227226,-2.5,41.6051310757064));
#7381=CARTESIAN_POINT('',(29.2525276373731,-6.5,37.3694661350993));
#7382=CARTESIAN_POINT('',(29.3284458350469,-6.5,38.1852477434919));
#7383=CARTESIAN_POINT('',(29.2525276373731,-4.5,37.3694661350993));
#7384=CARTESIAN_POINT('Origin',(22.3743640879348,-4.5,36.8515390576026));
#7385=CARTESIAN_POINT('',(11.6914587751786,-2.5,36.047114171797));
#7386=CARTESIAN_POINT('',(29.5689942527814,-6.5,37.3932961339159));
#7387=CARTESIAN_POINT('Origin',(22.1907831020815,-4.5,26.534454790004));
#7388=CARTESIAN_POINT('',(22.1907831020815,-2.5,26.534454790004));
#7389=CARTESIAN_POINT('',(9.97043327249462,-2.5,36.1567564233319));
#7390=CARTESIAN_POINT('',(22.1907831020815,-6.5,26.534454790004));
#7391=CARTESIAN_POINT('',(22.439614333362,-6.5,26.3385251156033));
#7392=CARTESIAN_POINT('',(22.1907831020815,-4.5,26.534454790004));
#7393=CARTESIAN_POINT('Origin',(22.140815160637,-4.5,26.4454738972255));
#7394=CARTESIAN_POINT('',(22.140815160637,-2.5,26.4454738972255));
#7395=CARTESIAN_POINT('',(24.2237158126922,-2.5,30.1546192858673));
#7396=CARTESIAN_POINT('',(22.140815160637,-6.5,26.4454738972255));
#7397=CARTESIAN_POINT('',(22.541978158155,-6.5,27.1598487671307));
#7398=CARTESIAN_POINT('',(22.140815160637,-4.5,26.4454738972255));
#7399=CARTESIAN_POINT('Origin',(15.6466401722657,-4.5,28.7699251208132));
#7400=CARTESIAN_POINT('',(15.6466401722657,-2.5,28.7699251208132));
#7401=CARTESIAN_POINT('',(5.56013147171207,-2.5,32.3801754655778));
#7402=CARTESIAN_POINT('',(15.6466401722657,-6.5,28.7699251208132));
#7403=CARTESIAN_POINT('',(22.439614333362,-6.5,26.3385251156033));
#7404=CARTESIAN_POINT('',(15.6466401722657,-4.5,28.7699251208132));
#7405=CARTESIAN_POINT('Origin',(0.,-4.5,48.6364583401654));
#7406=CARTESIAN_POINT('',(13.2184823984455,-6.5,27.0779747683097));
#7407=CARTESIAN_POINT('Origin',(0.,-6.5,48.6364583401654));
#7408=CARTESIAN_POINT('',(13.2184823984455,-2.5,27.0779747683097));
#7409=CARTESIAN_POINT('',(13.2184823984455,-4.5,27.0779747683097));
#7410=CARTESIAN_POINT('Origin',(0.,-2.5,48.6364583401654));
#7411=CARTESIAN_POINT('Origin',(30.2362881000144,-4.5,56.8032384613577));
#7412=CARTESIAN_POINT('',(30.2362881000144,-2.5,56.8032384613577));
#7413=CARTESIAN_POINT('',(24.5880719834211,-2.5,54.5460443640832));
#7414=CARTESIAN_POINT('',(15.7929555278825,-2.5,51.0312558824666));
#7415=CARTESIAN_POINT('',(24.5880719834211,-6.5,54.5460443640832));
#7416=CARTESIAN_POINT('',(24.5880719834211,-4.5,54.5460443640832));
#7417=CARTESIAN_POINT('',(30.2362881000144,-6.5,56.8032384613577));
#7418=CARTESIAN_POINT('',(30.5303837910408,-6.5,56.9207677917012));
#7419=CARTESIAN_POINT('',(30.2362881000144,-4.5,56.8032384613577));
#7420=CARTESIAN_POINT('Origin',(30.2883638428897,-4.5,56.7154745083027));
#7421=CARTESIAN_POINT('',(30.2883638428897,-2.5,56.7154745083027));
#7422=CARTESIAN_POINT('',(28.1176000360236,-2.5,60.3738920808626));
#7423=CARTESIAN_POINT('',(30.2883638428897,-6.5,56.7154745083027));
#7424=CARTESIAN_POINT('',(29.8702785564856,-6.5,57.4200792901642));
#7425=CARTESIAN_POINT('',(30.2883638428897,-4.5,56.7154745083027));
#7426=CARTESIAN_POINT('Origin',(25.0282425392193,-4.5,52.2535796035455));
#7427=CARTESIAN_POINT('',(16.8584196763548,-2.5,45.3235320057556));
#7428=CARTESIAN_POINT('',(30.5303837910408,-6.5,56.9207677917012));
#7429=CARTESIAN_POINT('Origin',(0.,-4.5,48.6364583401654));
#7430=CARTESIAN_POINT('',(23.7292735925589,-2.5,57.3782010500299));
#7431=CARTESIAN_POINT('Origin',(0.,-2.5,48.6364583401654));
#7432=CARTESIAN_POINT('',(23.7292735925589,-6.5,57.3782010500299));
#7433=CARTESIAN_POINT('',(23.7292735925589,-4.5,57.3782010500299));
#7434=CARTESIAN_POINT('Origin',(0.,-6.5,48.6364583401654));
#7435=CARTESIAN_POINT('Origin',(17.1105963211311,-4.5,22.403713360841));
#7436=CARTESIAN_POINT('',(17.1105963211311,-2.5,22.403713360841));
#7437=CARTESIAN_POINT('',(7.15787945733662,-2.5,34.3564982124716));
#7438=CARTESIAN_POINT('',(17.1105963211311,-6.5,22.403713360841));
#7439=CARTESIAN_POINT('',(17.3132539231097,-6.5,22.1603302978897));
#7440=CARTESIAN_POINT('',(17.1105963211311,-4.5,22.403713360841));
#7441=CARTESIAN_POINT('Origin',(17.0432201312255,-4.5,22.327065833251));
#7442=CARTESIAN_POINT('',(17.0432201312255,-2.5,22.327065833251));
#7443=CARTESIAN_POINT('',(19.8517790958416,-2.5,25.5220980995497));
#7444=CARTESIAN_POINT('',(17.0432201312255,-6.5,22.327065833251));
#7445=CARTESIAN_POINT('',(17.5841436418306,-6.5,22.9424234211658));
#7446=CARTESIAN_POINT('',(17.0432201312255,-4.5,22.327065833251));
#7447=CARTESIAN_POINT('Origin',(11.1742390317241,-4.5,25.9509371229247));
#7448=CARTESIAN_POINT('',(2.05875799995238,-2.5,31.5793979140848));
#7449=CARTESIAN_POINT('',(17.3132539231097,-6.5,22.1603302978897));
#7450=CARTESIAN_POINT('Origin',(4.57790069807404,-4.5,42.4313271208406));
#7451=CARTESIAN_POINT('',(13.6784299900821,-2.5,32.3241653975668));
#7452=CARTESIAN_POINT('',(4.57790069807404,-2.5,42.4313271208406));
#7453=CARTESIAN_POINT('',(2.010271039483,-2.5,45.2829687531184));
#7454=CARTESIAN_POINT('',(13.6784299900821,-6.5,32.3241653975668));
#7455=CARTESIAN_POINT('',(13.6784299900821,-4.5,32.3241653975668));
#7456=CARTESIAN_POINT('',(4.57790069807404,-6.5,42.4313271208406));
#7457=CARTESIAN_POINT('',(13.6784299900821,-6.5,32.3241653975668));
#7458=CARTESIAN_POINT('',(4.57790069807404,-4.5,42.4313271208406));
#7459=CARTESIAN_POINT('Origin',(14.7931472282982,-4.5,33.3278613071051));
#7460=CARTESIAN_POINT('',(5.69261793629013,-2.5,43.4350230303789));
#7461=CARTESIAN_POINT('',(14.7931472282982,-2.5,33.3278613071051));
#7462=CARTESIAN_POINT('',(7.67525292370313,-2.5,41.2330838010198));
#7463=CARTESIAN_POINT('',(5.69261793629014,-6.5,43.4350230303789));
#7464=CARTESIAN_POINT('',(5.69261793629013,-4.5,43.4350230303789));
#7465=CARTESIAN_POINT('',(14.7931472282982,-6.5,33.3278613071051));
#7466=CARTESIAN_POINT('',(5.69261793629014,-6.5,43.4350230303789));
#7467=CARTESIAN_POINT('',(14.7931472282982,-4.5,33.3278613071051));
#7468=CARTESIAN_POINT('Origin',(0.,-4.5,48.6364583401654));
#7469=CARTESIAN_POINT('',(7.28764508722295,-2.5,28.6344440135681));
#7470=CARTESIAN_POINT('Origin',(0.,-2.5,48.6364583401654));
#7471=CARTESIAN_POINT('',(7.28764508722295,-6.5,28.6344440135681));
#7472=CARTESIAN_POINT('',(7.28764508722295,-4.5,28.6344440135681));
#7473=CARTESIAN_POINT('Origin',(0.,-6.5,48.6364583401654));
#7474=CARTESIAN_POINT('Origin',(0.,-4.5,48.6364583401654));
#7475=CARTESIAN_POINT('',(19.1306748574635,-6.5,39.2979559154323));
#7476=CARTESIAN_POINT('Origin',(0.,-6.5,48.6364583401654));
#7477=CARTESIAN_POINT('',(19.1306748574635,-2.5,39.2979559154323));
#7478=CARTESIAN_POINT('',(19.1306748574635,-4.5,39.2979559154323));
#7479=CARTESIAN_POINT('Origin',(0.,-2.5,48.6364583401654));
#7480=CARTESIAN_POINT('Origin',(0.,-4.5,48.6364583401654));
#7481=CARTESIAN_POINT('',(3.08485092071416,-6.5,41.5693144299684));
#7482=CARTESIAN_POINT('Origin',(0.,-6.5,48.6364583401654));
#7483=CARTESIAN_POINT('',(3.08485092071416,-2.5,41.5693144299684));
#7484=CARTESIAN_POINT('',(3.08485092071416,-4.5,41.5693144299684));
#7485=CARTESIAN_POINT('Origin',(0.,-2.5,48.6364583401654));
#7486=CARTESIAN_POINT('Origin',(0.,-4.5,48.6364583401654));
#7487=CARTESIAN_POINT('',(6.70597463025744,-2.5,44.8297888629439));
#7488=CARTESIAN_POINT('Origin',(0.,-2.5,48.6364583401654));
#7489=CARTESIAN_POINT('',(6.70597463025745,-6.5,44.8297888629439));
#7490=CARTESIAN_POINT('',(6.70597463025744,-4.5,44.8297888629439));
#7491=CARTESIAN_POINT('Origin',(0.,-6.5,48.6364583401654));
#7492=CARTESIAN_POINT('Origin',(6.70597463025745,-4.5,44.8297888629439));
#7493=CARTESIAN_POINT('',(3.2004610739753,-2.5,46.3905440549387));
#7494=CARTESIAN_POINT('',(19.1306748574635,-6.5,39.2979559154323));
#7495=CARTESIAN_POINT('Origin',(19.7407798220772,-4.5,40.6682741018962));
#7496=CARTESIAN_POINT('',(7.31607959487115,-2.5,46.2001070494078));
#7497=CARTESIAN_POINT('',(19.7407798220772,-2.5,40.6682741018962));
#7498=CARTESIAN_POINT('',(10.022916152192,-2.5,44.9949457676468));
#7499=CARTESIAN_POINT('',(7.31607959487115,-6.5,46.2001070494078));
#7500=CARTESIAN_POINT('',(7.31607959487115,-4.5,46.2001070494078));
#7501=CARTESIAN_POINT('',(19.7407798220772,-6.5,40.6682741018962));
#7502=CARTESIAN_POINT('',(7.31607959487115,-6.5,46.2001070494078));
#7503=CARTESIAN_POINT('',(19.7407798220772,-4.5,40.6682741018962));
#7504=CARTESIAN_POINT('Origin',(0.,-4.5,48.6364583401654));
#7505=CARTESIAN_POINT('',(21.2750522452644,-6.5,47.8864583401654));
#7506=CARTESIAN_POINT('Origin',(0.,-6.5,48.6364583401654));
#7507=CARTESIAN_POINT('',(21.2750522452644,-2.5,47.8864583401654));
#7508=CARTESIAN_POINT('',(21.2750522452644,-4.5,47.8864583401654));
#7509=CARTESIAN_POINT('Origin',(0.,-2.5,48.6364583401654));
#7510=CARTESIAN_POINT('Origin',(0.,-4.5,48.6364583401654));
#7511=CARTESIAN_POINT('',(7.67452462700238,-2.5,47.8864583401654));
#7512=CARTESIAN_POINT('Origin',(0.,-2.5,48.6364583401654));
#7513=CARTESIAN_POINT('',(7.67452462700238,-6.5,47.8864583401654));
#7514=CARTESIAN_POINT('',(7.67452462700238,-4.5,47.8864583401654));
#7515=CARTESIAN_POINT('Origin',(0.,-6.5,48.6364583401654));
#7516=CARTESIAN_POINT('Origin',(1.65826614627142,-4.5,41.1057889384059));
#7517=CARTESIAN_POINT('',(5.86106031278022,-2.5,28.1709185220056));
#7518=CARTESIAN_POINT('',(1.65826614627142,-2.5,41.1057889384059));
#7519=CARTESIAN_POINT('',(0.472486879525025,-2.5,44.7552422663951));
#7520=CARTESIAN_POINT('',(5.86106031278022,-6.5,28.1709185220056));
#7521=CARTESIAN_POINT('',(5.86106031278022,-4.5,28.1709185220056));
#7522=CARTESIAN_POINT('',(1.65826614627142,-6.5,41.1057889384059));
#7523=CARTESIAN_POINT('',(5.86106031278022,-6.5,28.1709185220056));
#7524=CARTESIAN_POINT('',(1.65826614627142,-4.5,41.1057889384059));
#7525=CARTESIAN_POINT('Origin',(7.28764508722295,-4.5,28.6344440135681));
#7526=CARTESIAN_POINT('',(4.00046873722216,-2.5,38.7513325497573));
#7527=CARTESIAN_POINT('',(3.08485092071416,-6.5,41.5693144299684));
#7528=CARTESIAN_POINT('Origin',(0.,-4.5,48.6364583401654));
#7529=CARTESIAN_POINT('',(-1.47795709561032,-2.5,27.3995567096953));
#7530=CARTESIAN_POINT('Origin',(0.,-2.5,48.6364583401654));
#7531=CARTESIAN_POINT('',(-1.47795709561032,-6.5,27.3995567096953));
#7532=CARTESIAN_POINT('',(-1.47795709561032,-4.5,27.3995567096953));
#7533=CARTESIAN_POINT('Origin',(0.,-6.5,48.6364583401654));
#7534=CARTESIAN_POINT('Origin',(0.,-4.5,48.6364583401654));
#7535=CARTESIAN_POINT('',(-0.0563148440441186,-6.5,40.9255792146178));
#7536=CARTESIAN_POINT('Origin',(0.,-6.5,48.6364583401654));
#7537=CARTESIAN_POINT('',(-0.0563148440441168,-2.5,40.9255792146178));
#7538=CARTESIAN_POINT('',(-0.0563148440441168,-4.5,40.9255792146178));
#7539=CARTESIAN_POINT('Origin',(0.,-2.5,48.6364583401654));
#7540=CARTESIAN_POINT('Origin',(19.6613580057765,-4.5,73.0159664767883));
#7541=CARTESIAN_POINT('',(19.6613580057765,-2.5,73.0159664767883));
#7542=CARTESIAN_POINT('',(16.4186005814896,-2.5,67.8699199573963));
#7543=CARTESIAN_POINT('',(11.3691427358738,-2.5,59.8567565993746));
#7544=CARTESIAN_POINT('',(16.4186005814896,-6.5,67.8699199573963));
#7545=CARTESIAN_POINT('',(16.4186005814896,-4.5,67.8699199573963));
#7546=CARTESIAN_POINT('',(19.6613580057765,-6.5,73.0159664767883));
#7547=CARTESIAN_POINT('',(19.8302044107015,-6.5,73.2839148123218));
#7548=CARTESIAN_POINT('',(19.6613580057765,-4.5,73.0159664767883));
#7549=CARTESIAN_POINT('Origin',(19.7550745240459,-4.5,72.9755733009377));
#7550=CARTESIAN_POINT('',(19.7550745240459,-2.5,72.9755733009377));
#7551=CARTESIAN_POINT('',(15.8485258176388,-2.5,74.6593523377723));
#7552=CARTESIAN_POINT('',(19.7550745240459,-6.5,72.9755733009377));
#7553=CARTESIAN_POINT('',(19.0026801227739,-6.5,73.2998661782326));
#7554=CARTESIAN_POINT('',(19.7550745240459,-4.5,72.9755733009377));
#7555=CARTESIAN_POINT('Origin',(18.1221830191981,-4.5,66.2740027683071));
#7556=CARTESIAN_POINT('',(18.1221830191981,-2.5,66.2740027683071));
#7557=CARTESIAN_POINT('',(15.5860372577735,-2.5,55.8653750972342));
#7558=CARTESIAN_POINT('',(18.1221830191981,-6.5,66.2740027683071));
#7559=CARTESIAN_POINT('',(19.8302044107015,-6.5,73.2839148123218));
#7560=CARTESIAN_POINT('',(18.1221830191981,-4.5,66.2740027683071));
#7561=CARTESIAN_POINT('Origin',(0.,-4.5,48.6364583401654));
#7562=CARTESIAN_POINT('',(14.0591181563592,-2.5,69.6563938182185));
#7563=CARTESIAN_POINT('Origin',(0.,-2.5,48.6364583401654));
#7564=CARTESIAN_POINT('',(14.0591181563592,-6.5,69.6563938182185));
#7565=CARTESIAN_POINT('',(14.0591181563592,-4.5,69.6563938182185));
#7566=CARTESIAN_POINT('Origin',(0.,-6.5,48.6364583401654));
#7567=CARTESIAN_POINT('Origin',(0.,-4.5,48.6364583401654));
#7568=CARTESIAN_POINT('',(20.0586762913077,-6.5,64.0360036671066));
#7569=CARTESIAN_POINT('Origin',(0.,-6.5,48.6364583401654));
#7570=CARTESIAN_POINT('',(20.0586762913077,-2.5,64.0360036671066));
#7571=CARTESIAN_POINT('',(20.0586762913077,-4.5,64.0360036671066));
#7572=CARTESIAN_POINT('Origin',(0.,-2.5,48.6364583401654));
#7573=CARTESIAN_POINT('Origin',(1.57645741831176,-4.5,79.9165510130336));
#7574=CARTESIAN_POINT('',(1.57645741831176,-2.5,79.9165510130336));
#7575=CARTESIAN_POINT('',(1.97778180513783,-2.5,73.8472669342436));
#7576=CARTESIAN_POINT('',(2.60270384171029,-2.5,64.396484745176));
#7577=CARTESIAN_POINT('',(1.97778180513783,-6.5,73.8472669342436));
#7578=CARTESIAN_POINT('',(1.97778180513783,-4.5,73.8472669342436));
#7579=CARTESIAN_POINT('',(1.57645741831176,-6.5,79.9165510130336));
#7580=CARTESIAN_POINT('',(1.55556094933236,-6.5,80.2325711968123));
#7581=CARTESIAN_POINT('',(1.57645741831176,-4.5,79.9165510130336));
#7582=CARTESIAN_POINT('Origin',(1.67601818730369,-4.5,79.9389574346486));
#7583=CARTESIAN_POINT('',(1.67601818730369,-2.5,79.9389574346486));
#7584=CARTESIAN_POINT('',(-2.47414659150375,-2.5,79.0049515732318));
#7585=CARTESIAN_POINT('',(1.67601818730369,-6.5,79.9389574346486));
#7586=CARTESIAN_POINT('',(0.876703759504667,-6.5,79.7590695505599));
#7587=CARTESIAN_POINT('',(1.67601818730369,-4.5,79.9389574346486));
#7588=CARTESIAN_POINT('Origin',(4.29406553618938,-4.5,73.5574834396049));
#7589=CARTESIAN_POINT('',(4.29406553618938,-2.5,73.5574834396049));
#7590=CARTESIAN_POINT('',(8.3603183566449,-2.5,63.6460176893561));
#7591=CARTESIAN_POINT('',(4.29406553618938,-6.5,73.5574834396049));
#7592=CARTESIAN_POINT('',(1.55556094933236,-6.5,80.2325711968123));
#7593=CARTESIAN_POINT('',(4.29406553618938,-4.5,73.5574834396049));
#7594=CARTESIAN_POINT('Origin',(0.,-4.5,48.6364583401654));
#7595=CARTESIAN_POINT('',(-0.981142563718944,-2.5,73.9056856751205));
#7596=CARTESIAN_POINT('Origin',(0.,-2.5,48.6364583401654));
#7597=CARTESIAN_POINT('',(-0.981142563718944,-6.5,73.9056856751205));
#7598=CARTESIAN_POINT('',(-0.981142563718944,-4.5,73.9056856751205));
#7599=CARTESIAN_POINT('Origin',(0.,-6.5,48.6364583401654));
#7600=CARTESIAN_POINT('Origin',(0.,-4.5,48.6364583401654));
#7601=CARTESIAN_POINT('',(7.17618436914825,-6.5,72.8851463198474));
#7602=CARTESIAN_POINT('Origin',(0.,-6.5,48.6364583401654));
#7603=CARTESIAN_POINT('',(7.17618436914825,-2.5,72.8851463198474));
#7604=CARTESIAN_POINT('',(7.17618436914825,-4.5,72.8851463198474));
#7605=CARTESIAN_POINT('Origin',(0.,-2.5,48.6364583401654));
#7606=CARTESIAN_POINT('Origin',(8.04550499793291,-4.5,78.9052420115192));
#7607=CARTESIAN_POINT('',(8.04550499793291,-2.5,78.9052420115191));
#7608=CARTESIAN_POINT('',(5.82252225538788,-2.5,63.5109577993001));
#7609=CARTESIAN_POINT('',(8.04550499793291,-6.5,78.9052420115191));
#7610=CARTESIAN_POINT('',(8.09076945767885,-6.5,79.2187010162633));
#7611=CARTESIAN_POINT('',(8.04550499793291,-4.5,78.9052420115191));
#7612=CARTESIAN_POINT('Origin',(8.14754868225272,-4.5,78.9064589512426));
#7613=CARTESIAN_POINT('',(8.14754868225272,-2.5,78.9064589512426));
#7614=CARTESIAN_POINT('',(3.89388422333141,-2.5,78.8557311351607));
#7615=CARTESIAN_POINT('',(8.14754868225272,-6.5,78.9064589512426));
#7616=CARTESIAN_POINT('',(7.32830039833067,-6.5,78.8966888631989));
#7617=CARTESIAN_POINT('',(8.14754868225272,-4.5,78.9064589512426));
#7618=CARTESIAN_POINT('Origin',(9.38160236695365,-4.5,72.1201128228977));
#7619=CARTESIAN_POINT('',(9.38160236695366,-2.5,72.1201128228977));
#7620=CARTESIAN_POINT('',(11.2982882046428,-2.5,61.5798148803432));
#7621=CARTESIAN_POINT('',(9.38160236695365,-6.5,72.1201128228977));
#7622=CARTESIAN_POINT('',(8.09076945767885,-6.5,79.2187010162633));
#7623=CARTESIAN_POINT('',(9.38160236695366,-4.5,72.1201128228977));
#7624=CARTESIAN_POINT('Origin',(0.,-4.5,48.6364583401654));
#7625=CARTESIAN_POINT('',(12.0609532410738,-6.5,70.8632416826245));
#7626=CARTESIAN_POINT('Origin',(0.,-6.5,48.6364583401654));
#7627=CARTESIAN_POINT('',(12.0609532410738,-2.5,70.8632416826245));
#7628=CARTESIAN_POINT('',(12.0609532410738,-4.5,70.8632416826245));
#7629=CARTESIAN_POINT('Origin',(0.,-2.5,48.6364583401654));
#7630=CARTESIAN_POINT('Origin',(14.162925402528,-4.5,76.5710419178277));
#7631=CARTESIAN_POINT('',(14.162925402528,-2.5,76.5710419178277));
#7632=CARTESIAN_POINT('',(8.78786850694337,-2.5,61.9753438512926));
#7633=CARTESIAN_POINT('',(14.162925402528,-6.5,76.5710419178277));
#7634=CARTESIAN_POINT('',(14.2723725169055,-6.5,76.8682400808869));
#7635=CARTESIAN_POINT('',(14.162925402528,-4.5,76.5710419178277));
#7636=CARTESIAN_POINT('Origin',(14.262992203511,-4.5,76.5510161895543));
#7637=CARTESIAN_POINT('',(14.262992203511,-2.5,76.5510161895543));
#7638=CARTESIAN_POINT('',(10.0917336126774,-2.5,77.385783467789));
#7639=CARTESIAN_POINT('',(14.262992203511,-6.5,76.5510161895543));
#7640=CARTESIAN_POINT('',(13.4596151446628,-6.5,76.7117908972851));
#7641=CARTESIAN_POINT('',(14.262992203511,-4.5,76.5510161895543));
#7642=CARTESIAN_POINT('Origin',(14.0591181563592,-4.5,69.6563938182185));
#7643=CARTESIAN_POINT('',(13.7424686428958,-2.5,58.9479252814089));
#7644=CARTESIAN_POINT('',(14.2723725169055,-6.5,76.8682400808869));
#7645=CARTESIAN_POINT('Origin',(24.3004949185093,-4.5,68.3953895443191));
#7646=CARTESIAN_POINT('',(24.3004949185093,-2.5,68.3953895443191));
#7647=CARTESIAN_POINT('',(13.4535308720469,-2.5,57.2477884725646));
#7648=CARTESIAN_POINT('',(24.3004949185093,-6.5,68.3953895443191));
#7649=CARTESIAN_POINT('',(24.5213612158718,-6.5,68.6223774243054));
#7650=CARTESIAN_POINT('',(24.3004949185093,-4.5,68.3953895443191));
#7651=CARTESIAN_POINT('Origin',(24.383765292515,-4.5,68.3363942965038));
#7652=CARTESIAN_POINT('',(24.383765292515,-2.5,68.3363942965038));
#7653=CARTESIAN_POINT('',(20.912661394705,-2.5,70.7955958683606));
#7654=CARTESIAN_POINT('',(24.383765292515,-6.5,68.3363942965038));
#7655=CARTESIAN_POINT('',(23.7152367945438,-6.5,68.8100321884952));
#7656=CARTESIAN_POINT('',(24.383765292515,-4.5,68.3363942965038));
#7657=CARTESIAN_POINT('Origin',(21.3932215242158,-4.5,62.1207663925577));
#7658=CARTESIAN_POINT('',(21.3932215242158,-2.5,62.1207663925577));
#7659=CARTESIAN_POINT('',(16.7484212543818,-2.5,52.4668865625843));
#7660=CARTESIAN_POINT('',(21.3932215242158,-6.5,62.1207663925577));
#7661=CARTESIAN_POINT('',(24.5213612158718,-6.5,68.6223774243054));
#7662=CARTESIAN_POINT('',(21.3932215242158,-4.5,62.1207663925577));
#7663=CARTESIAN_POINT('Origin',(0.,-4.5,48.6364583401654));
#7664=CARTESIAN_POINT('',(22.8220915949877,-6.5,59.5290533508125));
#7665=CARTESIAN_POINT('Origin',(0.,-6.5,48.6364583401654));
#7666=CARTESIAN_POINT('',(22.8220915949877,-2.5,59.5290533508125));
#7667=CARTESIAN_POINT('',(22.8220915949877,-4.5,59.5290533508125));
#7668=CARTESIAN_POINT('Origin',(0.,-2.5,48.6364583401654));
#7669=CARTESIAN_POINT('Origin',(27.8775835965913,-4.5,62.9112525043571));
#7670=CARTESIAN_POINT('',(27.8775835965913,-2.5,62.9112525043571));
#7671=CARTESIAN_POINT('',(14.9499351519079,-2.5,54.2624638972222));
#7672=CARTESIAN_POINT('',(27.8775835965913,-6.5,62.9112525043571));
#7673=CARTESIAN_POINT('',(28.1408168693625,-6.5,63.087359469232));
#7674=CARTESIAN_POINT('',(27.8775835965913,-4.5,62.9112525043571));
#7675=CARTESIAN_POINT('Origin',(27.9467685114137,-4.5,62.8362335599973));
#7676=CARTESIAN_POINT('',(27.9467685114137,-2.5,62.8362335599973));
#7677=CARTESIAN_POINT('',(25.0628133187395,-2.5,65.9633787576275));
#7678=CARTESIAN_POINT('',(27.9467685114137,-6.5,62.8362335599973));
#7679=CARTESIAN_POINT('',(27.3913238200603,-6.5,63.4385162180383));
#7680=CARTESIAN_POINT('',(27.9467685114137,-4.5,62.8362335599973));
#7681=CARTESIAN_POINT('Origin',(23.7292735925589,-4.5,57.3782010500299));
#7682=CARTESIAN_POINT('',(17.1788188743319,-2.5,48.9009899341809));
#7683=CARTESIAN_POINT('',(28.1408168693625,-6.5,63.087359469232));
#7684=CARTESIAN_POINT('Origin',(-3.18774326066286,-4.5,55.6577916291187));
#7685=CARTESIAN_POINT('',(-9.98800706979388,-2.5,67.4361940514055));
#7686=CARTESIAN_POINT('',(-3.18774326066286,-2.5,55.6577916291187));
#7687=CARTESIAN_POINT('',(-1.26911210391227,-2.5,52.3346249846421));
#7688=CARTESIAN_POINT('',(-9.98800706979389,-6.5,67.4361940514055));
#7689=CARTESIAN_POINT('',(-9.98800706979388,-4.5,67.4361940514055));
#7690=CARTESIAN_POINT('',(-3.18774326066286,-6.5,55.6577916291187));
#7691=CARTESIAN_POINT('',(-9.98800706979389,-6.5,67.4361940514055));
#7692=CARTESIAN_POINT('',(-3.18774326066286,-4.5,55.6577916291187));
#7693=CARTESIAN_POINT('Origin',(-11.2870451754705,-4.5,66.6861940514055));
#7694=CARTESIAN_POINT('',(-4.48678136633952,-2.5,54.9077916291187));
#7695=CARTESIAN_POINT('',(-11.2870451754705,-2.5,66.6861940514055));
#7696=CARTESIAN_POINT('',(-5.96828211415444,-2.5,57.4738261957855));
#7697=CARTESIAN_POINT('',(-4.48678136633952,-6.5,54.9077916291187));
#7698=CARTESIAN_POINT('',(-4.48678136633952,-4.5,54.9077916291187));
#7699=CARTESIAN_POINT('',(-11.2870451754705,-6.5,66.6861940514055));
#7700=CARTESIAN_POINT('',(-4.48678136633952,-6.5,54.9077916291187));
#7701=CARTESIAN_POINT('',(-11.2870451754705,-4.5,66.6861940514055));
#7702=CARTESIAN_POINT('Origin',(0.,-4.5,48.6364583401654));
#7703=CARTESIAN_POINT('',(-2.96973993866275,-2.5,69.7165672757341));
#7704=CARTESIAN_POINT('Origin',(0.,-2.5,48.6364583401654));
#7705=CARTESIAN_POINT('',(-2.96973993866275,-6.5,69.7165672757341));
#7706=CARTESIAN_POINT('',(-2.96973993866275,-4.5,69.7165672757341));
#7707=CARTESIAN_POINT('Origin',(0.,-6.5,48.6364583401654));
#7708=CARTESIAN_POINT('Origin',(0.,-4.5,48.6364583401654));
#7709=CARTESIAN_POINT('',(-16.7710398834144,-6.5,61.7483830374649));
#7710=CARTESIAN_POINT('Origin',(0.,-6.5,48.6364583401654));
#7711=CARTESIAN_POINT('',(-16.7710398834144,-2.5,61.7483830374649));
#7712=CARTESIAN_POINT('',(-16.7710398834144,-4.5,61.7483830374649));
#7713=CARTESIAN_POINT('Origin',(0.,-2.5,48.6364583401654));
#7714=CARTESIAN_POINT('Origin',(0.,-4.5,48.6364583401654));
#7715=CARTESIAN_POINT('',(-1.54809768709653,-6.5,56.1905447708115));
#7716=CARTESIAN_POINT('Origin',(0.,-6.5,48.6364583401654));
#7717=CARTESIAN_POINT('',(-1.54809768709653,-2.5,56.1905447708115));
#7718=CARTESIAN_POINT('',(-1.54809768709653,-4.5,56.1905447708115));
#7719=CARTESIAN_POINT('Origin',(0.,-2.5,48.6364583401654));
#7720=CARTESIAN_POINT('Origin',(0.,-4.5,48.6364583401654));
#7721=CARTESIAN_POINT('',(-5.76798190777462,-2.5,53.754193480054));
#7722=CARTESIAN_POINT('Origin',(0.,-2.5,48.6364583401654));
#7723=CARTESIAN_POINT('',(-5.76798190777462,-6.5,53.754193480054));
#7724=CARTESIAN_POINT('',(-5.76798190777462,-4.5,53.754193480054));
#7725=CARTESIAN_POINT('Origin',(0.,-6.5,48.6364583401654));
#7726=CARTESIAN_POINT('Origin',(-5.76798190777462,-4.5,53.754193480054));
#7727=CARTESIAN_POINT('',(-2.66357148427763,-2.5,51.4987072830003));
#7728=CARTESIAN_POINT('',(-16.7710398834144,-6.5,61.7483830374649));
#7729=CARTESIAN_POINT('Origin',(-17.6527177618532,-4.5,60.5348575459025));
#7730=CARTESIAN_POINT('',(-6.64965978621333,-2.5,52.5406679884916));
#7731=CARTESIAN_POINT('',(-17.6527177618531,-2.5,60.5348575459025));
#7732=CARTESIAN_POINT('',(-9.04677835053625,-2.5,54.2822765701433));
#7733=CARTESIAN_POINT('',(-6.64965978621333,-6.5,52.5406679884916));
#7734=CARTESIAN_POINT('',(-6.64965978621333,-4.5,52.5406679884916));
#7735=CARTESIAN_POINT('',(-17.6527177618532,-6.5,60.5348575459025));
#7736=CARTESIAN_POINT('',(-6.64965978621333,-6.5,52.5406679884916));
#7737=CARTESIAN_POINT('',(-17.6527177618531,-4.5,60.5348575459025));
#7738=CARTESIAN_POINT('Origin',(0.,-4.5,48.6364583401654));
#7739=CARTESIAN_POINT('',(-20.6542075410784,-6.5,53.7934011252648));
#7740=CARTESIAN_POINT('Origin',(0.,-6.5,48.6364583401654));
#7741=CARTESIAN_POINT('',(-20.6542075410784,-2.5,53.7934011252648));
#7742=CARTESIAN_POINT('',(-20.6542075410784,-4.5,53.7934011252648));
#7743=CARTESIAN_POINT('Origin',(0.,-2.5,48.6364583401654));
#7744=CARTESIAN_POINT('Origin',(0.,-4.5,48.6364583401654));
#7745=CARTESIAN_POINT('',(-7.35088408256156,-2.5,50.9656924321383));
#7746=CARTESIAN_POINT('Origin',(0.,-2.5,48.6364583401654));
#7747=CARTESIAN_POINT('',(-7.35088408256156,-6.5,50.9656924321383));
#7748=CARTESIAN_POINT('',(-7.35088408256156,-4.5,50.9656924321383));
#7749=CARTESIAN_POINT('Origin',(0.,-6.5,48.6364583401654));
#7750=CARTESIAN_POINT('Origin',(3.08485092071416,-4.5,55.7036022503624));
#7751=CARTESIAN_POINT('',(7.28764508722295,-2.5,68.6384726667627));
#7752=CARTESIAN_POINT('',(3.08485092071415,-2.5,55.7036022503624));
#7753=CARTESIAN_POINT('',(1.89907165396776,-2.5,52.0541489223733));
#7754=CARTESIAN_POINT('',(7.28764508722294,-6.5,68.6384726667627));
#7755=CARTESIAN_POINT('',(7.28764508722295,-4.5,68.6384726667627));
#7756=CARTESIAN_POINT('',(3.08485092071416,-6.5,55.7036022503624));
#7757=CARTESIAN_POINT('',(7.28764508722294,-6.5,68.6384726667627));
#7758=CARTESIAN_POINT('',(3.08485092071415,-4.5,55.7036022503624));
#7759=CARTESIAN_POINT('Origin',(5.86106031278021,-4.5,69.1019981583252));
#7760=CARTESIAN_POINT('',(1.65826614627142,-2.5,56.1671277419249));
#7761=CARTESIAN_POINT('',(5.86106031278021,-2.5,69.1019981583252));
#7762=CARTESIAN_POINT('',(2.57388396277942,-2.5,58.9851096221359));
#7763=CARTESIAN_POINT('',(1.65826614627142,-6.5,56.1671277419249));
#7764=CARTESIAN_POINT('',(1.65826614627142,-4.5,56.1671277419249));
#7765=CARTESIAN_POINT('',(5.86106031278021,-6.5,69.1019981583252));
#7766=CARTESIAN_POINT('',(1.65826614627142,-6.5,56.1671277419249));
#7767=CARTESIAN_POINT('',(5.86106031278021,-4.5,69.1019981583252));
#7768=CARTESIAN_POINT('Origin',(0.,-4.5,48.6364583401654));
#7769=CARTESIAN_POINT('',(13.6784299900821,-2.5,64.948751282764));
#7770=CARTESIAN_POINT('Origin',(0.,-2.5,48.6364583401654));
#7771=CARTESIAN_POINT('',(13.6784299900821,-6.5,64.948751282764));
#7772=CARTESIAN_POINT('',(13.6784299900821,-4.5,64.948751282764));
#7773=CARTESIAN_POINT('Origin',(0.,-6.5,48.6364583401654));
#7774=CARTESIAN_POINT('Origin',(0.,-4.5,48.6364583401654));
#7775=CARTESIAN_POINT('',(-1.47795709561033,-6.5,69.8733599706355));
#7776=CARTESIAN_POINT('Origin',(0.,-6.5,48.6364583401654));
#7777=CARTESIAN_POINT('',(-1.47795709561034,-2.5,69.8733599706355));
#7778=CARTESIAN_POINT('',(-1.47795709561034,-4.5,69.8733599706355));
#7779=CARTESIAN_POINT('Origin',(0.,-2.5,48.6364583401654));
#7780=CARTESIAN_POINT('Origin',(0.,-4.5,48.6364583401654));
#7781=CARTESIAN_POINT('',(4.57790069807404,-6.5,54.8415895594902));
#7782=CARTESIAN_POINT('Origin',(0.,-6.5,48.6364583401654));
#7783=CARTESIAN_POINT('',(4.57790069807404,-2.5,54.8415895594902));
#7784=CARTESIAN_POINT('',(4.57790069807404,-4.5,54.8415895594902));
#7785=CARTESIAN_POINT('Origin',(0.,-2.5,48.6364583401654));
#7786=CARTESIAN_POINT('Origin',(0.,-4.5,48.6364583401654));
#7787=CARTESIAN_POINT('',(-0.0563148440441184,-2.5,56.347337465713));
#7788=CARTESIAN_POINT('Origin',(0.,-2.5,48.6364583401654));
#7789=CARTESIAN_POINT('',(-0.0563148440441186,-6.5,56.347337465713));
#7790=CARTESIAN_POINT('',(-0.0563148440441184,-4.5,56.347337465713));
#7791=CARTESIAN_POINT('Origin',(0.,-6.5,48.6364583401654));
#7792=CARTESIAN_POINT('Origin',(7.31607959487115,-4.5,51.0728096309229));
#7793=CARTESIAN_POINT('',(19.7407798220772,-2.5,56.6046425784346));
#7794=CARTESIAN_POINT('',(7.31607959487115,-2.5,51.0728096309229));
#7795=CARTESIAN_POINT('',(3.810566038589,-2.5,49.5120544389282));
#7796=CARTESIAN_POINT('',(19.7407798220772,-6.5,56.6046425784346));
#7797=CARTESIAN_POINT('',(19.7407798220772,-4.5,56.6046425784346));
#7798=CARTESIAN_POINT('',(7.31607959487115,-6.5,51.0728096309229));
#7799=CARTESIAN_POINT('',(19.7407798220772,-6.5,56.6046425784346));
#7800=CARTESIAN_POINT('',(7.31607959487115,-4.5,51.0728096309229));
#7801=CARTESIAN_POINT('Origin',(19.1306748574635,-4.5,57.9749607648985));
#7802=CARTESIAN_POINT('',(6.70597463025744,-2.5,52.4431278173869));
#7803=CARTESIAN_POINT('',(19.1306748574635,-2.5,57.9749607648985));
#7804=CARTESIAN_POINT('',(9.41281118757831,-2.5,53.6482890991479));
#7805=CARTESIAN_POINT('',(6.70597463025744,-6.5,52.4431278173869));
#7806=CARTESIAN_POINT('',(6.70597463025744,-4.5,52.4431278173869));
#7807=CARTESIAN_POINT('',(19.1306748574635,-6.5,57.9749607648985));
#7808=CARTESIAN_POINT('',(6.70597463025744,-6.5,52.4431278173869));
#7809=CARTESIAN_POINT('',(19.1306748574635,-4.5,57.9749607648985));
#7810=CARTESIAN_POINT('Origin',(0.,-4.5,48.6364583401654));
#7811=CARTESIAN_POINT('',(21.2750522452644,-2.5,49.3864583401654));
#7812=CARTESIAN_POINT('Origin',(0.,-2.5,48.6364583401654));
#7813=CARTESIAN_POINT('',(21.2750522452644,-6.5,49.3864583401654));
#7814=CARTESIAN_POINT('',(21.2750522452644,-4.5,49.3864583401654));
#7815=CARTESIAN_POINT('Origin',(0.,-6.5,48.6364583401654));
#7816=CARTESIAN_POINT('Origin',(0.,-4.5,48.6364583401654));
#7817=CARTESIAN_POINT('',(14.7931472282982,-6.5,63.9450553732257));
#7818=CARTESIAN_POINT('Origin',(0.,-6.5,48.6364583401654));
#7819=CARTESIAN_POINT('',(14.7931472282982,-2.5,63.9450553732257));
#7820=CARTESIAN_POINT('',(14.7931472282982,-4.5,63.9450553732257));
#7821=CARTESIAN_POINT('Origin',(0.,-2.5,48.6364583401654));
#7822=CARTESIAN_POINT('Origin',(0.,-4.5,48.6364583401654));
#7823=CARTESIAN_POINT('',(7.67452462700238,-6.5,49.3864583401654));
#7824=CARTESIAN_POINT('Origin',(0.,-6.5,48.6364583401654));
#7825=CARTESIAN_POINT('',(7.67452462700238,-2.5,49.3864583401654));
#7826=CARTESIAN_POINT('',(7.67452462700238,-4.5,49.3864583401654));
#7827=CARTESIAN_POINT('Origin',(0.,-2.5,48.6364583401654));
#7828=CARTESIAN_POINT('Origin',(0.,-4.5,48.6364583401654));
#7829=CARTESIAN_POINT('',(5.69261793629013,-2.5,53.8378936499519));
#7830=CARTESIAN_POINT('Origin',(0.,-2.5,48.6364583401654));
#7831=CARTESIAN_POINT('',(5.69261793629014,-6.5,53.8378936499519));
#7832=CARTESIAN_POINT('',(5.69261793629013,-4.5,53.8378936499519));
#7833=CARTESIAN_POINT('Origin',(0.,-6.5,48.6364583401654));
#7834=CARTESIAN_POINT('Origin',(-7.35088408256156,-4.5,50.9656924321383));
#7835=CARTESIAN_POINT('',(-3.59747515722412,-2.5,50.167880736427));
#7836=CARTESIAN_POINT('',(-20.6542075410784,-6.5,53.7934011252648));
#7837=CARTESIAN_POINT('Origin',(-20.9660750773051,-4.5,52.3261797241641));
#7838=CARTESIAN_POINT('',(-7.66275161878819,-2.5,49.4984710310376));
#7839=CARTESIAN_POINT('',(-20.9660750773051,-2.5,52.3261797241641));
#7840=CARTESIAN_POINT('',(-10.5610044227092,-2.5,50.1145136818896));
#7841=CARTESIAN_POINT('',(-7.6627516187882,-6.5,49.4984710310376));
#7842=CARTESIAN_POINT('',(-7.66275161878819,-4.5,49.4984710310376));
#7843=CARTESIAN_POINT('',(-20.9660750773051,-6.5,52.3261797241641));
#7844=CARTESIAN_POINT('',(-7.6627516187882,-6.5,49.4984710310376));
#7845=CARTESIAN_POINT('',(-20.9660750773051,-4.5,52.3261797241641));
#7846=CARTESIAN_POINT('Origin',(0.,-4.5,48.6364583401654));
#7847=CARTESIAN_POINT('',(-20.9660750773051,-6.5,44.9467369561667));
#7848=CARTESIAN_POINT('Origin',(0.,-6.5,48.6364583401654));
#7849=CARTESIAN_POINT('',(-20.9660750773051,-2.5,44.9467369561667));
#7850=CARTESIAN_POINT('',(-20.9660750773051,-4.5,44.9467369561667));
#7851=CARTESIAN_POINT('Origin',(0.,-2.5,48.6364583401654));
#7852=CARTESIAN_POINT('Origin',(0.,-4.5,48.6364583401654));
#7853=CARTESIAN_POINT('',(-7.6627516187882,-2.5,47.7744456492932));
#7854=CARTESIAN_POINT('Origin',(0.,-2.5,48.6364583401654));
#7855=CARTESIAN_POINT('',(-7.6627516187882,-6.5,47.7744456492932));
#7856=CARTESIAN_POINT('',(-7.6627516187882,-4.5,47.7744456492932));
#7857=CARTESIAN_POINT('Origin',(0.,-6.5,48.6364583401654));
#7858=CARTESIAN_POINT('Origin',(5.69261793629014,-4.5,53.8378936499519));
#7859=CARTESIAN_POINT('',(3.12498827769909,-2.5,50.9862520176741));
#7860=CARTESIAN_POINT('',(14.7931472282982,-6.5,63.9450553732257));
#7861=CARTESIAN_POINT('Origin',(13.6784299900821,-4.5,64.948751282764));
#7862=CARTESIAN_POINT('',(6.56053568548703,-2.5,57.0435287888493));
#7863=CARTESIAN_POINT('',(4.57790069807404,-6.5,54.8415895594902));
#7864=CARTESIAN_POINT('Origin',(-7.6627516187882,-4.5,47.7744456492932));
#7865=CARTESIAN_POINT('',(-3.90934269345076,-2.5,48.5722573450045));
#7866=CARTESIAN_POINT('',(-20.9660750773051,-6.5,44.9467369561667));
#7867=CARTESIAN_POINT('Origin',(-20.6542075410784,-4.5,43.4795155550659));
#7868=CARTESIAN_POINT('',(-7.35088408256156,-2.5,46.3072242481924));
#7869=CARTESIAN_POINT('',(-20.6542075410784,-2.5,43.4795155550659));
#7870=CARTESIAN_POINT('',(-10.2491368864826,-2.5,45.6911815973405));
#7871=CARTESIAN_POINT('',(-7.35088408256156,-6.5,46.3072242481924));
#7872=CARTESIAN_POINT('',(-7.35088408256156,-4.5,46.3072242481924));
#7873=CARTESIAN_POINT('',(-20.6542075410784,-6.5,43.4795155550659));
#7874=CARTESIAN_POINT('',(-7.35088408256156,-6.5,46.3072242481924));
#7875=CARTESIAN_POINT('',(-20.6542075410784,-4.5,43.4795155550659));
#7876=CARTESIAN_POINT('Origin',(0.,-4.5,48.6364583401654));
#7877=CARTESIAN_POINT('',(-17.6527177618531,-6.5,36.7380591344283));
#7878=CARTESIAN_POINT('Origin',(0.,-6.5,48.6364583401654));
#7879=CARTESIAN_POINT('',(-17.6527177618531,-2.5,36.7380591344283));
#7880=CARTESIAN_POINT('',(-17.6527177618531,-4.5,36.7380591344283));
#7881=CARTESIAN_POINT('Origin',(0.,-2.5,48.6364583401654));
#7882=CARTESIAN_POINT('Origin',(0.,-4.5,48.6364583401654));
#7883=CARTESIAN_POINT('',(-6.64965978621333,-2.5,44.7322486918392));
#7884=CARTESIAN_POINT('Origin',(0.,-2.5,48.6364583401654));
#7885=CARTESIAN_POINT('',(-6.64965978621333,-6.5,44.7322486918392));
#7886=CARTESIAN_POINT('',(-6.64965978621333,-4.5,44.7322486918392));
#7887=CARTESIAN_POINT('Origin',(0.,-6.5,48.6364583401654));
#7888=CARTESIAN_POINT('Origin',(-0.0563148440441186,-4.5,56.347337465713));
#7889=CARTESIAN_POINT('',(0.344788288741045,-2.5,52.5310960766646));
#7890=CARTESIAN_POINT('',(-1.47795709561033,-6.5,69.8733599706355));
#7891=CARTESIAN_POINT('Origin',(-2.96973993866275,-4.5,69.7165672757341));
#7892=CARTESIAN_POINT('',(-1.85781568009448,-2.5,59.1373146342244));
#7893=CARTESIAN_POINT('',(-1.54809768709653,-6.5,56.1905447708115));
#7894=CARTESIAN_POINT('Origin',(-1.57645741831176,-4.5,17.3563656672972));
#7895=CARTESIAN_POINT('',(-1.57645741831176,-2.5,17.3563656672972));
#7896=CARTESIAN_POINT('',(-1.97778180513782,-2.5,23.4256497460872));
#7897=CARTESIAN_POINT('',(-2.60270384171029,-2.5,32.8764319351548));
#7898=CARTESIAN_POINT('',(-1.97778180513782,-6.5,23.4256497460872));
#7899=CARTESIAN_POINT('',(-1.97778180513782,-4.5,23.4256497460872));
#7900=CARTESIAN_POINT('',(-1.57645741831176,-6.5,17.3563656672972));
#7901=CARTESIAN_POINT('',(-1.55556094933235,-6.5,17.0403454835185));
#7902=CARTESIAN_POINT('',(-1.57645741831176,-4.5,17.3563656672972));
#7903=CARTESIAN_POINT('Origin',(-1.67601818730369,-4.5,17.3339592456822));
#7904=CARTESIAN_POINT('',(-1.67601818730369,-2.5,17.3339592456822));
#7905=CARTESIAN_POINT('',(2.47414659150376,-2.5,18.267965107099));
#7906=CARTESIAN_POINT('',(-1.67601818730369,-6.5,17.3339592456822));
#7907=CARTESIAN_POINT('',(-0.87670375950466,-6.5,17.5138471297709));
#7908=CARTESIAN_POINT('',(-1.67601818730369,-4.5,17.3339592456822));
#7909=CARTESIAN_POINT('Origin',(-4.29406553618937,-4.5,23.7154332407259));
#7910=CARTESIAN_POINT('',(-4.29406553618937,-2.5,23.7154332407259));
#7911=CARTESIAN_POINT('',(-8.3603183566449,-2.5,33.6268989909746));
#7912=CARTESIAN_POINT('',(-4.29406553618937,-6.5,23.7154332407259));
#7913=CARTESIAN_POINT('',(-1.55556094933235,-6.5,17.0403454835185));
#7914=CARTESIAN_POINT('',(-4.29406553618937,-4.5,23.7154332407259));
#7915=CARTESIAN_POINT('Origin',(0.,-4.5,48.6364583401654));
#7916=CARTESIAN_POINT('',(0.981142563718935,-2.5,23.3672310052103));
#7917=CARTESIAN_POINT('Origin',(0.,-2.5,48.6364583401654));
#7918=CARTESIAN_POINT('',(0.981142563718941,-6.5,23.3672310052103));
#7919=CARTESIAN_POINT('',(0.981142563718935,-4.5,23.3672310052103));
#7920=CARTESIAN_POINT('Origin',(0.,-6.5,48.6364583401654));
#7921=CARTESIAN_POINT('Origin',(0.,-4.5,48.6364583401654));
#7922=CARTESIAN_POINT('',(-7.17618436914824,-6.5,24.3877703604834));
#7923=CARTESIAN_POINT('Origin',(0.,-6.5,48.6364583401654));
#7924=CARTESIAN_POINT('',(-7.17618436914824,-2.5,24.3877703604834));
#7925=CARTESIAN_POINT('',(-7.17618436914824,-4.5,24.3877703604834));
#7926=CARTESIAN_POINT('Origin',(0.,-2.5,48.6364583401654));
#7927=CARTESIAN_POINT('Origin',(-8.04550499793289,-4.5,18.3676746688116));
#7928=CARTESIAN_POINT('',(-8.04550499793289,-2.5,18.3676746688116));
#7929=CARTESIAN_POINT('',(-5.82252225538787,-2.5,33.7619588810307));
#7930=CARTESIAN_POINT('',(-8.04550499793289,-6.5,18.3676746688116));
#7931=CARTESIAN_POINT('',(-8.09076945767883,-6.5,18.0542156640675));
#7932=CARTESIAN_POINT('',(-8.04550499793289,-4.5,18.3676746688116));
#7933=CARTESIAN_POINT('Origin',(-8.14754868225271,-4.5,18.3664577290881));
#7934=CARTESIAN_POINT('',(-8.14754868225271,-2.5,18.3664577290881));
#7935=CARTESIAN_POINT('',(-3.8938842233314,-2.5,18.4171855451701));
#7936=CARTESIAN_POINT('',(-8.14754868225271,-6.5,18.3664577290881));
#7937=CARTESIAN_POINT('',(-7.32830039833065,-6.5,18.3762278171319));
#7938=CARTESIAN_POINT('',(-8.14754868225271,-4.5,18.3664577290881));
#7939=CARTESIAN_POINT('Origin',(-9.38160236695364,-4.5,25.1528038574331));
#7940=CARTESIAN_POINT('',(-9.38160236695365,-2.5,25.1528038574331));
#7941=CARTESIAN_POINT('',(-11.2982882046428,-2.5,35.6931017999876));
#7942=CARTESIAN_POINT('',(-9.38160236695364,-6.5,25.1528038574331));
#7943=CARTESIAN_POINT('',(-8.09076945767883,-6.5,18.0542156640675));
#7944=CARTESIAN_POINT('',(-9.38160236695365,-4.5,25.1528038574331));
#7945=CARTESIAN_POINT('Origin',(0.,-4.5,48.6364583401654));
#7946=CARTESIAN_POINT('',(-12.0609532410738,-6.5,26.4096749977063));
#7947=CARTESIAN_POINT('Origin',(0.,-6.5,48.6364583401654));
#7948=CARTESIAN_POINT('',(-12.0609532410738,-2.5,26.4096749977063));
#7949=CARTESIAN_POINT('',(-12.0609532410738,-4.5,26.4096749977063));
#7950=CARTESIAN_POINT('Origin',(0.,-2.5,48.6364583401654));
#7951=CARTESIAN_POINT('Origin',(-19.6613580057765,-4.5,24.2569502035424));
#7952=CARTESIAN_POINT('',(-19.6613580057765,-2.5,24.2569502035424));
#7953=CARTESIAN_POINT('',(-16.4186005814896,-2.5,29.4029967229345));
#7954=CARTESIAN_POINT('',(-11.3691427358738,-2.5,37.4161600809562));
#7955=CARTESIAN_POINT('',(-16.4186005814896,-6.5,29.4029967229345));
#7956=CARTESIAN_POINT('',(-16.4186005814896,-4.5,29.4029967229345));
#7957=CARTESIAN_POINT('',(-19.6613580057765,-6.5,24.2569502035424));
#7958=CARTESIAN_POINT('',(-19.8302044107015,-6.5,23.989001868009));
#7959=CARTESIAN_POINT('',(-19.6613580057765,-4.5,24.2569502035424));
#7960=CARTESIAN_POINT('Origin',(-19.7550745240459,-4.5,24.2973433793931));
#7961=CARTESIAN_POINT('',(-19.7550745240459,-2.5,24.2973433793931));
#7962=CARTESIAN_POINT('',(-15.8485258176388,-2.5,22.6135643425585));
#7963=CARTESIAN_POINT('',(-19.7550745240459,-6.5,24.2973433793931));
#7964=CARTESIAN_POINT('',(-19.0026801227739,-6.5,23.9730505020982));
#7965=CARTESIAN_POINT('',(-19.7550745240459,-4.5,24.2973433793931));
#7966=CARTESIAN_POINT('Origin',(-18.1221830191981,-4.5,30.9989139120237));
#7967=CARTESIAN_POINT('',(-18.1221830191981,-2.5,30.9989139120237));
#7968=CARTESIAN_POINT('',(-15.5860372577735,-2.5,41.4075415830966));
#7969=CARTESIAN_POINT('',(-18.1221830191981,-6.5,30.9989139120237));
#7970=CARTESIAN_POINT('',(-19.8302044107015,-6.5,23.989001868009));
#7971=CARTESIAN_POINT('',(-18.1221830191981,-4.5,30.9989139120237));
#7972=CARTESIAN_POINT('Origin',(0.,-4.5,48.6364583401654));
#7973=CARTESIAN_POINT('',(-14.0591181563592,-2.5,27.6165228621123));
#7974=CARTESIAN_POINT('Origin',(0.,-2.5,48.6364583401654));
#7975=CARTESIAN_POINT('',(-14.0591181563592,-6.5,27.6165228621123));
#7976=CARTESIAN_POINT('',(-14.0591181563592,-4.5,27.6165228621123));
#7977=CARTESIAN_POINT('Origin',(0.,-6.5,48.6364583401654));
#7978=CARTESIAN_POINT('Origin',(0.,-4.5,48.6364583401654));
#7979=CARTESIAN_POINT('',(-20.0586762913076,-6.5,33.2369130132242));
#7980=CARTESIAN_POINT('Origin',(0.,-6.5,48.6364583401654));
#7981=CARTESIAN_POINT('',(-20.0586762913077,-2.5,33.2369130132242));
#7982=CARTESIAN_POINT('',(-20.0586762913077,-4.5,33.2369130132242));
#7983=CARTESIAN_POINT('Origin',(0.,-2.5,48.6364583401654));
#7984=CARTESIAN_POINT('Origin',(-27.8775835965913,-4.5,34.3616641759737));
#7985=CARTESIAN_POINT('',(-27.8775835965913,-2.5,34.3616641759737));
#7986=CARTESIAN_POINT('',(-22.8220915949877,-2.5,37.7438633295183));
#7987=CARTESIAN_POINT('',(-14.9499351519079,-2.5,43.0104527831085));
#7988=CARTESIAN_POINT('',(-22.8220915949877,-6.5,37.7438633295183));
#7989=CARTESIAN_POINT('',(-22.8220915949877,-4.5,37.7438633295183));
#7990=CARTESIAN_POINT('',(-27.8775835965913,-6.5,34.3616641759737));
#7991=CARTESIAN_POINT('',(-28.1408168693625,-6.5,34.1855572110988));
#7992=CARTESIAN_POINT('',(-27.8775835965913,-4.5,34.3616641759737));
#7993=CARTESIAN_POINT('Origin',(-27.9467685114137,-4.5,34.4366831203335));
#7994=CARTESIAN_POINT('',(-27.9467685114137,-2.5,34.4366831203335));
#7995=CARTESIAN_POINT('',(-25.0628133187395,-2.5,31.3095379227032));
#7996=CARTESIAN_POINT('',(-27.9467685114137,-6.5,34.4366831203335));
#7997=CARTESIAN_POINT('',(-27.3913238200603,-6.5,33.8344004622925));
#7998=CARTESIAN_POINT('',(-27.9467685114137,-4.5,34.4366831203335));
#7999=CARTESIAN_POINT('Origin',(-23.7292735925589,-4.5,39.8947156303009));
#8000=CARTESIAN_POINT('',(-23.7292735925589,-2.5,39.8947156303009));
#8001=CARTESIAN_POINT('',(-17.1788188743319,-2.5,48.3719267461499));
#8002=CARTESIAN_POINT('',(-23.7292735925589,-6.5,39.8947156303009));
#8003=CARTESIAN_POINT('',(-28.1408168693625,-6.5,34.1855572110988));
#8004=CARTESIAN_POINT('',(-23.7292735925589,-4.5,39.8947156303009));
#8005=CARTESIAN_POINT('Origin',(0.,-4.5,48.6364583401654));
#8006=CARTESIAN_POINT('',(-21.3932215242158,-2.5,35.152150287773));
#8007=CARTESIAN_POINT('Origin',(0.,-2.5,48.6364583401654));
#8008=CARTESIAN_POINT('',(-21.3932215242158,-6.5,35.152150287773));
#8009=CARTESIAN_POINT('',(-21.3932215242158,-4.5,35.152150287773));
#8010=CARTESIAN_POINT('Origin',(0.,-6.5,48.6364583401654));
#8011=CARTESIAN_POINT('Origin',(0.,-4.5,48.6364583401654));
#8012=CARTESIAN_POINT('',(-24.5880719834211,-6.5,42.7268723162475));
#8013=CARTESIAN_POINT('Origin',(0.,-6.5,48.6364583401654));
#8014=CARTESIAN_POINT('',(-24.5880719834211,-2.5,42.7268723162476));
#8015=CARTESIAN_POINT('',(-24.5880719834211,-4.5,42.7268723162476));
#8016=CARTESIAN_POINT('Origin',(0.,-2.5,48.6364583401654));
#8017=CARTESIAN_POINT('Origin',(-24.3004949185092,-4.5,28.8775271360116));
#8018=CARTESIAN_POINT('',(-24.3004949185092,-2.5,28.8775271360116));
#8019=CARTESIAN_POINT('',(-13.4535308720469,-2.5,40.0251282077662));
#8020=CARTESIAN_POINT('',(-24.3004949185092,-6.5,28.8775271360116));
#8021=CARTESIAN_POINT('',(-24.5213612158718,-6.5,28.6505392560254));
#8022=CARTESIAN_POINT('',(-24.3004949185092,-4.5,28.8775271360116));
#8023=CARTESIAN_POINT('Origin',(-24.383765292515,-4.5,28.936522383827));
#8024=CARTESIAN_POINT('',(-24.383765292515,-2.5,28.936522383827));
#8025=CARTESIAN_POINT('',(-20.912661394705,-2.5,26.4773208119702));
#8026=CARTESIAN_POINT('',(-24.383765292515,-6.5,28.936522383827));
#8027=CARTESIAN_POINT('',(-23.7152367945438,-6.5,28.4628844918356));
#8028=CARTESIAN_POINT('',(-24.383765292515,-4.5,28.936522383827));
#8029=CARTESIAN_POINT('Origin',(-21.3932215242158,-4.5,35.152150287773));
#8030=CARTESIAN_POINT('',(-16.7484212543818,-2.5,44.8060301177464));
#8031=CARTESIAN_POINT('',(-24.5213612158718,-6.5,28.6505392560254));
#8032=CARTESIAN_POINT('Origin',(4.96148891517159,-4.5,17.7121468141248));
#8033=CARTESIAN_POINT('',(4.96148891517159,-2.5,17.7121468141248));
#8034=CARTESIAN_POINT('',(0.730865219008715,-2.5,32.679693768175));
#8035=CARTESIAN_POINT('',(4.96148891517159,-6.5,17.7121468141248));
#8036=CARTESIAN_POINT('',(5.04763303690956,-6.5,17.4073770497759));
#8037=CARTESIAN_POINT('',(4.96148891517159,-4.5,17.7121468141248));
#8038=CARTESIAN_POINT('Origin',(4.86876234485807,-4.5,17.6695301787609));
#8039=CARTESIAN_POINT('',(4.86876234485807,-2.5,17.6695301787609));
#8040=CARTESIAN_POINT('',(8.73404532801765,-2.5,19.4459935475112));
#8041=CARTESIAN_POINT('',(4.86876234485807,-6.5,17.6695301787609));
#8042=CARTESIAN_POINT('',(5.61320904050308,-6.5,18.0116738951621));
#8043=CARTESIAN_POINT('',(4.86876234485807,-4.5,17.6695301787609));
#8044=CARTESIAN_POINT('Origin',(0.981142563718943,-4.5,23.3672310052103));
#8045=CARTESIAN_POINT('',(-5.05696247920324,-2.5,32.216685949378));
#8046=CARTESIAN_POINT('',(5.04763303690956,-6.5,17.4073770497759));
#8047=CARTESIAN_POINT('Origin',(-14.162925402528,-4.5,20.7018747625031));
#8048=CARTESIAN_POINT('',(-14.162925402528,-2.5,20.7018747625031));
#8049=CARTESIAN_POINT('',(-8.78786850694337,-2.5,35.2975728290382));
#8050=CARTESIAN_POINT('',(-14.162925402528,-6.5,20.7018747625031));
#8051=CARTESIAN_POINT('',(-14.2723725169055,-6.5,20.4046765994439));
#8052=CARTESIAN_POINT('',(-14.162925402528,-4.5,20.7018747625031));
#8053=CARTESIAN_POINT('Origin',(-14.262992203511,-4.5,20.7219004907765));
#8054=CARTESIAN_POINT('',(-14.262992203511,-2.5,20.7219004907765));
#8055=CARTESIAN_POINT('',(-10.0917336126774,-2.5,19.8871332125418));
#8056=CARTESIAN_POINT('',(-14.262992203511,-6.5,20.7219004907765));
#8057=CARTESIAN_POINT('',(-13.4596151446628,-6.5,20.5611257830457));
#8058=CARTESIAN_POINT('',(-14.262992203511,-4.5,20.7219004907765));
#8059=CARTESIAN_POINT('Origin',(-14.0591181563592,-4.5,27.6165228621123));
#8060=CARTESIAN_POINT('',(-13.7424686428958,-2.5,38.3249913989219));
#8061=CARTESIAN_POINT('',(-14.2723725169055,-6.5,20.4046765994439));
#8062=CARTESIAN_POINT('Origin',(-30.2362881000144,-4.5,40.4696782189731));
#8063=CARTESIAN_POINT('',(-30.2362881000144,-2.5,40.4696782189731));
#8064=CARTESIAN_POINT('',(-15.7929555278825,-2.5,46.2416607978642));
#8065=CARTESIAN_POINT('',(-30.2362881000144,-6.5,40.4696782189731));
#8066=CARTESIAN_POINT('',(-30.5303837910408,-6.5,40.3521488886295));
#8067=CARTESIAN_POINT('',(-30.2362881000144,-4.5,40.4696782189731));
#8068=CARTESIAN_POINT('Origin',(-30.2883638428897,-4.5,40.557442172028));
#8069=CARTESIAN_POINT('',(-30.2883638428897,-2.5,40.557442172028));
#8070=CARTESIAN_POINT('',(-28.1176000360236,-2.5,36.8990245994682));
#8071=CARTESIAN_POINT('',(-30.2883638428897,-6.5,40.557442172028));
#8072=CARTESIAN_POINT('',(-29.8702785564856,-6.5,39.8528373901666));
#8073=CARTESIAN_POINT('',(-30.2883638428897,-4.5,40.557442172028));
#8074=CARTESIAN_POINT('Origin',(-25.0282425392193,-4.5,45.0193370767853));
#8075=CARTESIAN_POINT('',(-25.0282425392193,-2.5,45.0193370767853));
#8076=CARTESIAN_POINT('',(-16.8584196763548,-2.5,51.9493846745752));
#8077=CARTESIAN_POINT('',(-25.0282425392193,-6.5,45.0193370767853));
#8078=CARTESIAN_POINT('',(-30.5303837910408,-6.5,40.3521488886295));
#8079=CARTESIAN_POINT('',(-25.0282425392193,-4.5,45.0193370767853));
#8080=CARTESIAN_POINT('Origin',(0.,-4.5,48.6364583401654));
#8081=CARTESIAN_POINT('',(-25.2794356395192,-6.5,47.968158569562));
#8082=CARTESIAN_POINT('Origin',(0.,-6.5,48.6364583401654));
#8083=CARTESIAN_POINT('',(-25.2794356395192,-2.5,47.968158569562));
#8084=CARTESIAN_POINT('',(-25.2794356395192,-4.5,47.968158569562));
#8085=CARTESIAN_POINT('Origin',(0.,-2.5,48.6364583401654));
#8086=CARTESIAN_POINT('Origin',(-6.64965978621333,-4.5,44.7322486918392));
#8087=CARTESIAN_POINT('',(-3.54524936271634,-2.5,46.9877348888929));
#8088=CARTESIAN_POINT('',(-17.6527177618531,-6.5,36.7380591344283));
#8089=CARTESIAN_POINT('Origin',(-16.7710398834144,-4.5,35.5245336428659));
#8090=CARTESIAN_POINT('',(-5.76798190777462,-2.5,43.5187232002768));
#8091=CARTESIAN_POINT('',(-16.7710398834144,-2.5,35.5245336428659));
#8092=CARTESIAN_POINT('',(-8.16510047209754,-2.5,41.777114618625));
#8093=CARTESIAN_POINT('',(-5.76798190777462,-6.5,43.5187232002768));
#8094=CARTESIAN_POINT('',(-5.76798190777462,-4.5,43.5187232002768));
#8095=CARTESIAN_POINT('',(-16.7710398834144,-6.5,35.5245336428659));
#8096=CARTESIAN_POINT('',(-5.76798190777462,-6.5,43.5187232002768));
#8097=CARTESIAN_POINT('',(-16.7710398834144,-4.5,35.5245336428659));
#8098=CARTESIAN_POINT('Origin',(0.,-4.5,48.6364583401654));
#8099=CARTESIAN_POINT('',(-11.2870451754705,-6.5,30.5867226289253));
#8100=CARTESIAN_POINT('Origin',(0.,-6.5,48.6364583401654));
#8101=CARTESIAN_POINT('',(-11.2870451754705,-2.5,30.5867226289253));
#8102=CARTESIAN_POINT('',(-11.2870451754705,-4.5,30.5867226289253));
#8103=CARTESIAN_POINT('Origin',(0.,-2.5,48.6364583401654));
#8104=CARTESIAN_POINT('Origin',(0.,-4.5,48.6364583401654));
#8105=CARTESIAN_POINT('',(-4.48678136633952,-2.5,42.365125051212));
#8106=CARTESIAN_POINT('Origin',(0.,-2.5,48.6364583401654));
#8107=CARTESIAN_POINT('',(-4.48678136633952,-6.5,42.365125051212));
#8108=CARTESIAN_POINT('',(-4.48678136633952,-4.5,42.365125051212));
#8109=CARTESIAN_POINT('Origin',(0.,-6.5,48.6364583401654));
#8110=CARTESIAN_POINT('Origin',(-1.54809768709653,-4.5,41.0823719095192));
#8111=CARTESIAN_POINT('',(-2.96973993866273,-2.5,27.5563494045967));
#8112=CARTESIAN_POINT('',(-1.54809768709653,-2.5,41.0823719095192));
#8113=CARTESIAN_POINT('',(-1.14699455431137,-2.5,44.8986132985677));
#8114=CARTESIAN_POINT('',(-2.96973993866273,-6.5,27.5563494045967));
#8115=CARTESIAN_POINT('',(-2.96973993866273,-4.5,27.5563494045967));
#8116=CARTESIAN_POINT('',(-1.54809768709653,-6.5,41.0823719095192));
#8117=CARTESIAN_POINT('',(-2.96973993866273,-6.5,27.5563494045967));
#8118=CARTESIAN_POINT('',(-1.54809768709653,-4.5,41.0823719095192));
#8119=CARTESIAN_POINT('Origin',(-1.47795709561032,-4.5,27.3995567096953));
#8120=CARTESIAN_POINT('',(-0.366032837042061,-2.5,37.978809351205));
#8121=CARTESIAN_POINT('',(-0.0563148440441186,-6.5,40.9255792146178));
#8122=CARTESIAN_POINT('Origin',(0.,-4.5,48.6364583401654));
#8123=CARTESIAN_POINT('',(-9.98800706979387,-2.5,29.8367226289253));
#8124=CARTESIAN_POINT('Origin',(0.,-2.5,48.6364583401654));
#8125=CARTESIAN_POINT('',(-9.98800706979387,-6.5,29.8367226289253));
#8126=CARTESIAN_POINT('',(-9.98800706979387,-4.5,29.8367226289253));
#8127=CARTESIAN_POINT('Origin',(0.,-6.5,48.6364583401654));
#8128=CARTESIAN_POINT('Origin',(0.,-4.5,48.6364583401654));
#8129=CARTESIAN_POINT('',(-3.18774326066286,-6.5,41.615125051212));
#8130=CARTESIAN_POINT('Origin',(0.,-6.5,48.6364583401654));
#8131=CARTESIAN_POINT('',(-3.18774326066286,-2.5,41.615125051212));
#8132=CARTESIAN_POINT('',(-3.18774326066286,-4.5,41.615125051212));
#8133=CARTESIAN_POINT('Origin',(0.,-2.5,48.6364583401654));
#8134=CARTESIAN_POINT('Origin',(-4.48678136633952,-4.5,42.365125051212));
#8135=CARTESIAN_POINT('',(-2.56815020958893,-2.5,45.6882916956887));
#8136=CARTESIAN_POINT('',(-11.2870451754705,-6.5,30.5867226289253));
#8137=CARTESIAN_POINT('Origin',(-9.98800706979387,-4.5,29.8367226289253));
#8138=CARTESIAN_POINT('',(-4.66924400847777,-2.5,39.0490904845453));
#8139=CARTESIAN_POINT('',(-3.18774326066286,-6.5,41.615125051212));
#8140=CARTESIAN_POINT('Origin',(-29.2619838336808,-4.5,59.8018386620522));
#8141=CARTESIAN_POINT('',(-29.2619838336808,-2.5,59.8018386620522));
#8142=CARTESIAN_POINT('',(-23.3657356055148,-2.5,58.3080089112559));
#8143=CARTESIAN_POINT('',(-14.1843960910556,-2.5,55.9818927797566));
#8144=CARTESIAN_POINT('',(-23.3657356055148,-6.5,58.3080089112559));
#8145=CARTESIAN_POINT('',(-23.3657356055148,-4.5,58.3080089112559));
#8146=CARTESIAN_POINT('',(-29.2619838336808,-6.5,59.8018386620522));
#8147=CARTESIAN_POINT('',(-29.5689942527814,-6.5,59.8796205464148));
#8148=CARTESIAN_POINT('',(-29.2619838336808,-4.5,59.8018386620522));
#8149=CARTESIAN_POINT('Origin',(-29.2525276373731,-4.5,59.9034505452315));
#8150=CARTESIAN_POINT('',(-29.2525276373731,-2.5,59.9034505452315));
#8151=CARTESIAN_POINT('',(-29.6467067227226,-2.5,55.6677856046244));
#8152=CARTESIAN_POINT('',(-29.2525276373731,-6.5,59.9034505452315));
#8153=CARTESIAN_POINT('',(-29.3284458350469,-6.5,59.0876689368389));
#8154=CARTESIAN_POINT('',(-29.2525276373731,-4.5,59.9034505452315));
#8155=CARTESIAN_POINT('Origin',(-22.3743640879348,-4.5,60.4213776227282));
#8156=CARTESIAN_POINT('',(-22.3743640879347,-2.5,60.4213776227282));
#8157=CARTESIAN_POINT('',(-11.6914587751786,-2.5,61.2258025085338));
#8158=CARTESIAN_POINT('',(-22.3743640879347,-6.5,60.4213776227282));
#8159=CARTESIAN_POINT('',(-29.5689942527814,-6.5,59.8796205464148));
#8160=CARTESIAN_POINT('',(-22.3743640879347,-4.5,60.4213776227282));
#8161=CARTESIAN_POINT('Origin',(0.,-4.5,48.6364583401654));
#8162=CARTESIAN_POINT('',(-24.3356530447464,-2.5,55.511956992751));
#8163=CARTESIAN_POINT('Origin',(0.,-2.5,48.6364583401654));
#8164=CARTESIAN_POINT('',(-24.3356530447464,-6.5,55.5119569927511));
#8165=CARTESIAN_POINT('',(-24.3356530447464,-4.5,55.511956992751));
#8166=CARTESIAN_POINT('Origin',(0.,-6.5,48.6364583401654));
#8167=CARTESIAN_POINT('Origin',(0.,-4.5,48.6364583401654));
#8168=CARTESIAN_POINT('',(-20.8443097898499,-6.5,62.9546719235965));
#8169=CARTESIAN_POINT('Origin',(0.,-6.5,48.6364583401654));
#8170=CARTESIAN_POINT('',(-20.8443097898499,-2.5,62.9546719235965));
#8171=CARTESIAN_POINT('',(-20.8443097898499,-4.5,62.9546719235965));
#8172=CARTESIAN_POINT('Origin',(0.,-2.5,48.6364583401654));
#8173=CARTESIAN_POINT('Origin',(-26.3011261782795,-4.5,65.6417568488419));
#8174=CARTESIAN_POINT('',(-26.3011261782795,-2.5,65.6417568488419));
#8175=CARTESIAN_POINT('',(-12.3472313101976,-2.5,58.7704791881192));
#8176=CARTESIAN_POINT('',(-26.3011261782795,-6.5,65.6417568488419));
#8177=CARTESIAN_POINT('',(-26.5852559200301,-6.5,65.7816700677457));
#8178=CARTESIAN_POINT('',(-26.3011261782795,-4.5,65.6417568488419));
#8179=CARTESIAN_POINT('Origin',(-26.27075032411,-4.5,65.7391822148167));
#8180=CARTESIAN_POINT('',(-26.27075032411,-2.5,65.7391822148167));
#8181=CARTESIAN_POINT('',(-27.5369599102432,-2.5,61.6780311557697));
#8182=CARTESIAN_POINT('',(-26.27075032411,-6.5,65.7391822148167));
#8183=CARTESIAN_POINT('',(-26.5146200605557,-6.5,64.957011672687));
#8184=CARTESIAN_POINT('',(-26.27075032411,-4.5,65.7391822148167));
#8185=CARTESIAN_POINT('Origin',(-19.4352080563696,-4.5,64.8157407297404));
#8186=CARTESIAN_POINT('',(-19.4352080563695,-2.5,64.8157407297404));
#8187=CARTESIAN_POINT('',(-8.81850051768697,-2.5,63.3814860953406));
#8188=CARTESIAN_POINT('',(-19.4352080563696,-6.5,64.8157407297404));
#8189=CARTESIAN_POINT('',(-26.5852559200301,-6.5,65.7816700677457));
#8190=CARTESIAN_POINT('',(-19.4352080563695,-4.5,64.8157407297404));
#8191=CARTESIAN_POINT('Origin',(0.,-4.5,48.6364583401654));
#8192=CARTESIAN_POINT('',(-17.4118876142729,-6.5,66.9755602959296));
#8193=CARTESIAN_POINT('Origin',(0.,-6.5,48.6364583401654));
#8194=CARTESIAN_POINT('',(-17.4118876142729,-2.5,66.9755602959296));
#8195=CARTESIAN_POINT('',(-17.4118876142729,-4.5,66.9755602959296));
#8196=CARTESIAN_POINT('Origin',(0.,-2.5,48.6364583401654));
#8197=CARTESIAN_POINT('Origin',(-11.2825943751967,-4.5,77.8534479143798));
#8198=CARTESIAN_POINT('',(-11.2825943751967,-2.5,77.8534479143798));
#8199=CARTESIAN_POINT('',(-8.44736607249009,-2.5,72.4721143469408));
#8200=CARTESIAN_POINT('',(-4.03249196257662,-2.5,64.092573898288));
#8201=CARTESIAN_POINT('',(-8.44736607249009,-6.5,72.4721143469408));
#8202=CARTESIAN_POINT('',(-8.44736607249009,-4.5,72.4721143469408));
#8203=CARTESIAN_POINT('',(-11.2825943751967,-6.5,77.8534479143798));
#8204=CARTESIAN_POINT('',(-11.4302212382079,-6.5,78.1336473581494));
#8205=CARTESIAN_POINT('',(-11.2825943751967,-4.5,77.8534479143798));
#8206=CARTESIAN_POINT('Origin',(-11.2007545996357,-4.5,77.91441221203));
#8207=CARTESIAN_POINT('',(-11.2007545996357,-2.5,77.91441221203));
#8208=CARTESIAN_POINT('',(-14.6122243730978,-2.5,75.3731313095776));
#8209=CARTESIAN_POINT('',(-11.2007545996357,-6.5,77.91441221203));
#8210=CARTESIAN_POINT('',(-11.8577976702754,-6.5,77.4249659855108));
#8211=CARTESIAN_POINT('',(-11.2007545996357,-4.5,77.91441221203));
#8212=CARTESIAN_POINT('Origin',(-6.21347002554836,-4.5,73.1495014208928));
#8213=CARTESIAN_POINT('',(-6.21347002554835,-2.5,73.1495014208928));
#8214=CARTESIAN_POINT('',(1.53259307542215,-2.5,65.7488209282624));
#8215=CARTESIAN_POINT('',(-6.21347002554836,-6.5,73.1495014208928));
#8216=CARTESIAN_POINT('',(-11.4302212382079,-6.5,78.1336473581494));
#8217=CARTESIAN_POINT('',(-6.21347002554835,-4.5,73.1495014208928));
#8218=CARTESIAN_POINT('Origin',(0.,-4.5,48.6364583401654));
#8219=CARTESIAN_POINT('',(-11.1742390317241,-2.5,71.3219795574061));
#8220=CARTESIAN_POINT('Origin',(0.,-2.5,48.6364583401654));
#8221=CARTESIAN_POINT('',(-11.1742390317241,-6.5,71.3219795574061));
#8222=CARTESIAN_POINT('',(-11.1742390317241,-4.5,71.3219795574061));
#8223=CARTESIAN_POINT('Origin',(0.,-6.5,48.6364583401654));
#8224=CARTESIAN_POINT('Origin',(0.,-4.5,48.6364583401654));
#8225=CARTESIAN_POINT('',(-3.30705931420718,-6.5,73.707554238197));
#8226=CARTESIAN_POINT('Origin',(0.,-6.5,48.6364583401654));
#8227=CARTESIAN_POINT('',(-3.30705931420718,-2.5,73.707554238197));
#8228=CARTESIAN_POINT('',(-3.30705931420718,-4.5,73.707554238197));
#8229=CARTESIAN_POINT('Origin',(0.,-2.5,48.6364583401654));
#8230=CARTESIAN_POINT('Origin',(-22.1907831020815,-4.5,70.7384618903268));
#8231=CARTESIAN_POINT('',(-22.1907831020815,-2.5,70.7384618903268));
#8232=CARTESIAN_POINT('',(-9.97043327249461,-2.5,61.1161602569989));
#8233=CARTESIAN_POINT('',(-22.1907831020815,-6.5,70.7384618903268));
#8234=CARTESIAN_POINT('',(-22.439614333362,-6.5,70.9343915647275));
#8235=CARTESIAN_POINT('',(-22.1907831020815,-4.5,70.7384618903268));
#8236=CARTESIAN_POINT('Origin',(-22.140815160637,-4.5,70.8274427831053));
#8237=CARTESIAN_POINT('',(-22.140815160637,-2.5,70.8274427831053));
#8238=CARTESIAN_POINT('',(-24.2237158126922,-2.5,67.1182973944635));
#8239=CARTESIAN_POINT('',(-22.140815160637,-6.5,70.8274427831053));
#8240=CARTESIAN_POINT('',(-22.541978158155,-6.5,70.1130679132001));
#8241=CARTESIAN_POINT('',(-22.140815160637,-4.5,70.8274427831053));
#8242=CARTESIAN_POINT('Origin',(-15.6466401722657,-4.5,68.5029915595176));
#8243=CARTESIAN_POINT('',(-15.6466401722657,-2.5,68.5029915595176));
#8244=CARTESIAN_POINT('',(-5.56013147171207,-2.5,64.892741214753));
#8245=CARTESIAN_POINT('',(-15.6466401722657,-6.5,68.5029915595176));
#8246=CARTESIAN_POINT('',(-22.439614333362,-6.5,70.9343915647275));
#8247=CARTESIAN_POINT('',(-15.6466401722657,-4.5,68.5029915595176));
#8248=CARTESIAN_POINT('Origin',(0.,-4.5,48.6364583401654));
#8249=CARTESIAN_POINT('',(-13.2184823984455,-6.5,70.1949419120211));
#8250=CARTESIAN_POINT('Origin',(0.,-6.5,48.6364583401654));
#8251=CARTESIAN_POINT('',(-13.2184823984455,-2.5,70.1949419120211));
#8252=CARTESIAN_POINT('',(-13.2184823984455,-4.5,70.1949419120211));
#8253=CARTESIAN_POINT('Origin',(0.,-2.5,48.6364583401654));
#8254=CARTESIAN_POINT('Origin',(-31.2735217236592,-4.5,46.9346197418275));
#8255=CARTESIAN_POINT('',(-31.2735217236592,-2.5,46.9346197418275));
#8256=CARTESIAN_POINT('',(-15.94574796428,-2.5,49.577532956732));
#8257=CARTESIAN_POINT('',(-31.2735217236592,-6.5,46.9346197418275));
#8258=CARTESIAN_POINT('',(-31.5856264400152,-6.5,46.8808046417196));
#8259=CARTESIAN_POINT('',(-31.2735217236592,-4.5,46.9346197418275));
#8260=CARTESIAN_POINT('Origin',(-31.3062123347366,-4.5,47.0312929976909));
#8261=CARTESIAN_POINT('',(-31.3062123347366,-2.5,47.0312929976909));
#8262=CARTESIAN_POINT('',(-29.943512708519,-2.5,43.0014934531576));
#8263=CARTESIAN_POINT('',(-31.3062123347366,-6.5,47.0312929976909));
#8264=CARTESIAN_POINT('',(-31.0437587864934,-6.5,46.2551607020453));
#8265=CARTESIAN_POINT('',(-31.3062123347366,-4.5,47.0312929976909));
#8266=CARTESIAN_POINT('Origin',(-25.2333571880834,-4.5,50.302044079353));
#8267=CARTESIAN_POINT('',(-25.2333571880834,-2.5,50.302044079353));
#8268=CARTESIAN_POINT('',(-15.8012266428482,-2.5,55.3820518250025));
#8269=CARTESIAN_POINT('',(-25.2333571880834,-6.5,50.302044079353));
#8270=CARTESIAN_POINT('',(-31.5856264400152,-6.5,46.8808046417196));
#8271=CARTESIAN_POINT('',(-25.2333571880834,-4.5,50.302044079353));
#8272=CARTESIAN_POINT('Origin',(0.,-4.5,48.6364583401654));
#8273=CARTESIAN_POINT('',(-24.8659666539797,-6.5,53.2386527297099));
#8274=CARTESIAN_POINT('Origin',(0.,-6.5,48.6364583401654));
#8275=CARTESIAN_POINT('',(-24.8659666539797,-2.5,53.2386527297099));
#8276=CARTESIAN_POINT('',(-24.8659666539797,-4.5,53.2386527297099));
#8277=CARTESIAN_POINT('Origin',(0.,-2.5,48.6364583401654));
#8278=CARTESIAN_POINT('Origin',(-4.9614889151716,-4.5,79.5607698662059));
#8279=CARTESIAN_POINT('',(-4.9614889151716,-2.5,79.5607698662059));
#8280=CARTESIAN_POINT('',(-0.730865219008718,-2.5,64.5932229121558));
#8281=CARTESIAN_POINT('',(-4.9614889151716,-6.5,79.5607698662059));
#8282=CARTESIAN_POINT('',(-5.04763303690956,-6.5,79.8655396305548));
#8283=CARTESIAN_POINT('',(-4.9614889151716,-4.5,79.5607698662059));
#8284=CARTESIAN_POINT('Origin',(-4.86876234485807,-4.5,79.6033865015699));
#8285=CARTESIAN_POINT('',(-4.86876234485807,-2.5,79.6033865015699));
#8286=CARTESIAN_POINT('',(-8.73404532801766,-2.5,77.8269231328196));
#8287=CARTESIAN_POINT('',(-4.86876234485807,-6.5,79.6033865015699));
#8288=CARTESIAN_POINT('',(-5.61320904050309,-6.5,79.2612427851687));
#8289=CARTESIAN_POINT('',(-4.86876234485807,-4.5,79.6033865015699));
#8290=CARTESIAN_POINT('Origin',(-0.981142563718946,-4.5,73.9056856751205));
#8291=CARTESIAN_POINT('',(5.05696247920323,-2.5,65.0562307309528));
#8292=CARTESIAN_POINT('',(-5.04763303690956,-6.5,79.8655396305548));
#8293=CARTESIAN_POINT('Origin',(-17.1105963211311,-4.5,74.8692033194898));
#8294=CARTESIAN_POINT('',(-17.1105963211311,-2.5,74.8692033194898));
#8295=CARTESIAN_POINT('',(-7.15787945733663,-2.5,62.9164184678592));
#8296=CARTESIAN_POINT('',(-17.1105963211311,-6.5,74.8692033194898));
#8297=CARTESIAN_POINT('',(-17.3132539231097,-6.5,75.1125863824411));
#8298=CARTESIAN_POINT('',(-17.1105963211311,-4.5,74.8692033194898));
#8299=CARTESIAN_POINT('Origin',(-17.0432201312256,-4.5,74.9458508470798));
#8300=CARTESIAN_POINT('',(-17.0432201312256,-2.5,74.9458508470798));
#8301=CARTESIAN_POINT('',(-19.8517790958416,-2.5,71.7508185807811));
#8302=CARTESIAN_POINT('',(-17.0432201312256,-6.5,74.9458508470798));
#8303=CARTESIAN_POINT('',(-17.5841436418306,-6.5,74.330493259165));
#8304=CARTESIAN_POINT('',(-17.0432201312256,-4.5,74.9458508470798));
#8305=CARTESIAN_POINT('Origin',(-11.1742390317242,-4.5,71.3219795574061));
#8306=CARTESIAN_POINT('',(-2.05875799995239,-2.5,65.693518766246));
#8307=CARTESIAN_POINT('',(-17.3132539231097,-6.5,75.1125863824411));
#8308=CARTESIAN_POINT('Origin',(-30.9439523809731,-4.5,53.4739397777569));
#8309=CARTESIAN_POINT('',(-30.9439523809731,-2.5,53.4739397777569));
#8310=CARTESIAN_POINT('',(-15.4016346984504,-2.5,52.8722756390788));
#8311=CARTESIAN_POINT('',(-30.9439523809731,-6.5,53.4739397777569));
#8312=CARTESIAN_POINT('',(-31.2604256489094,-6.5,53.4861908859929));
#8313=CARTESIAN_POINT('',(-30.9439523809731,-4.5,53.4739397777569));
#8314=CARTESIAN_POINT('Origin',(-30.9558291236816,-4.5,53.5752972512578));
#8315=CARTESIAN_POINT('',(-30.9558291236816,-2.5,53.5752972512578));
#8316=CARTESIAN_POINT('',(-30.4607501907366,-2.5,49.3502373119707));
#8317=CARTESIAN_POINT('',(-30.9558291236816,-6.5,53.5752972512578));
#8318=CARTESIAN_POINT('',(-30.8604777930494,-6.5,52.7615581474436));
#8319=CARTESIAN_POINT('',(-30.9558291236816,-4.5,53.5752972512578));
#8320=CARTESIAN_POINT('Origin',(-24.3356530447464,-4.5,55.5119569927511));
#8321=CARTESIAN_POINT('',(-14.0534441823513,-2.5,58.5199041711936));
#8322=CARTESIAN_POINT('',(-31.2604256489094,-6.5,53.4861908859929));
#8323=CARTESIAN_POINT('Origin',(7.67452462700238,-4.5,47.8864583401654));
#8324=CARTESIAN_POINT('',(3.83726231350119,-2.5,47.8864583401654));
#8325=CARTESIAN_POINT('',(21.2750522452644,-6.5,47.8864583401654));
#8326=CARTESIAN_POINT('Origin',(21.2750522452644,-4.5,49.3864583401654));
#8327=CARTESIAN_POINT('',(10.6375261226322,-2.5,49.3864583401654));
#8328=CARTESIAN_POINT('',(7.67452462700238,-6.5,49.3864583401654));
#8329=CARTESIAN_POINT('Origin',(0.,-4.5,48.6364583401654));
#8330=CARTESIAN_POINT('',(-1.99137169252308,-2.5,48.6364583401654));
#8331=CARTESIAN_POINT('Origin',(0.,-2.5,48.6364583401654));
#8332=CARTESIAN_POINT('',(-1.99137169252308,-6.5,48.6364583401654));
#8333=CARTESIAN_POINT('',(-1.99137169252308,-4.5,48.6364583401654));
#8334=CARTESIAN_POINT('Origin',(0.,-6.5,48.6364583401654));
#8335=CARTESIAN_POINT('Origin',(0.,-2.5,48.6364583401654));
#8336=CARTESIAN_POINT('Origin',(0.,-6.5,48.6364583401654));
#8763=UNCERTAINTY_MEASURE_WITH_UNIT(LENGTH_MEASURE(0.01),#8780,
'DISTANCE_ACCURACY_VALUE',
'Maximum model space distance between geometric entities at asserted c
onnectivities');
#8770=UNCERTAINTY_MEASURE_WITH_UNIT(LENGTH_MEASURE(0.01),#8780,
'DISTANCE_ACCURACY_VALUE',
'Maximum model space distance between geometric entities at asserted c
onnectivities');
#8772=(
GEOMETRIC_REPRESENTATION_CONTEXT(3)
GLOBAL_UNCERTAINTY_ASSIGNED_CONTEXT((#8763))
GLOBAL_UNIT_ASSIGNED_CONTEXT((#8780,#8782,#8783))
REPRESENTATION_CONTEXT('','3D')
);
#8779=(
GEOMETRIC_REPRESENTATION_CONTEXT(3)
GLOBAL_UNCERTAINTY_ASSIGNED_CONTEXT((#8770))
GLOBAL_UNIT_ASSIGNED_CONTEXT((#8780,#8782,#8783))
REPRESENTATION_CONTEXT('','3D')
);
#8780=(
LENGTH_UNIT()
NAMED_UNIT(*)
SI_UNIT(.MILLI.,.METRE.)
);
#8782=(
NAMED_UNIT(*)
PLANE_ANGLE_UNIT()
SI_UNIT($,.RADIAN.)
);
#8783=(
NAMED_UNIT(*)
SI_UNIT($,.STERADIAN.)
SOLID_ANGLE_UNIT()
);
#8785=SHAPE_DEFINITION_REPRESENTATION(#8793,#8809);
#8793=PRODUCT_DEFINITION_SHAPE('',$,#8818);
#8809=SHAPE_REPRESENTATION('',(#5203),#8772);
#8816=PRODUCT_DEFINITION_CONTEXT('part definition',#8842,'design');
#8818=PRODUCT_DEFINITION('Wheel','Wheel',#8826,#8816);
#8826=PRODUCT_DEFINITION_FORMATION('',$,#8845);
#8842=APPLICATION_CONTEXT(
'Core Data for Automotive Mechanical Design Process');
#8843=PRODUCT_CONTEXT('part definition',#8842,'mechanical');
#8845=PRODUCT('Wheel','Wheel',$,(#8843));
#8853=PRESENTATION_STYLE_ASSIGNMENT((#8858));
#8858=SURFACE_STYLE_USAGE(.BOTH.,#8863);
#8863=SURFACE_SIDE_STYLE('',(#8868));
#8868=SURFACE_STYLE_FILL_AREA(#8873);
#8873=FILL_AREA_STYLE('Opaque(170,85,255)',(#8878));
#8878=FILL_AREA_STYLE_COLOUR('Opaque(170,85,255)',#8883);
#8883=COLOUR_RGB('Opaque(170,85,255)', 0.09019608, 0.27058824, 0.51372549);
ENDSEC;
END-ISO-10303-21;
